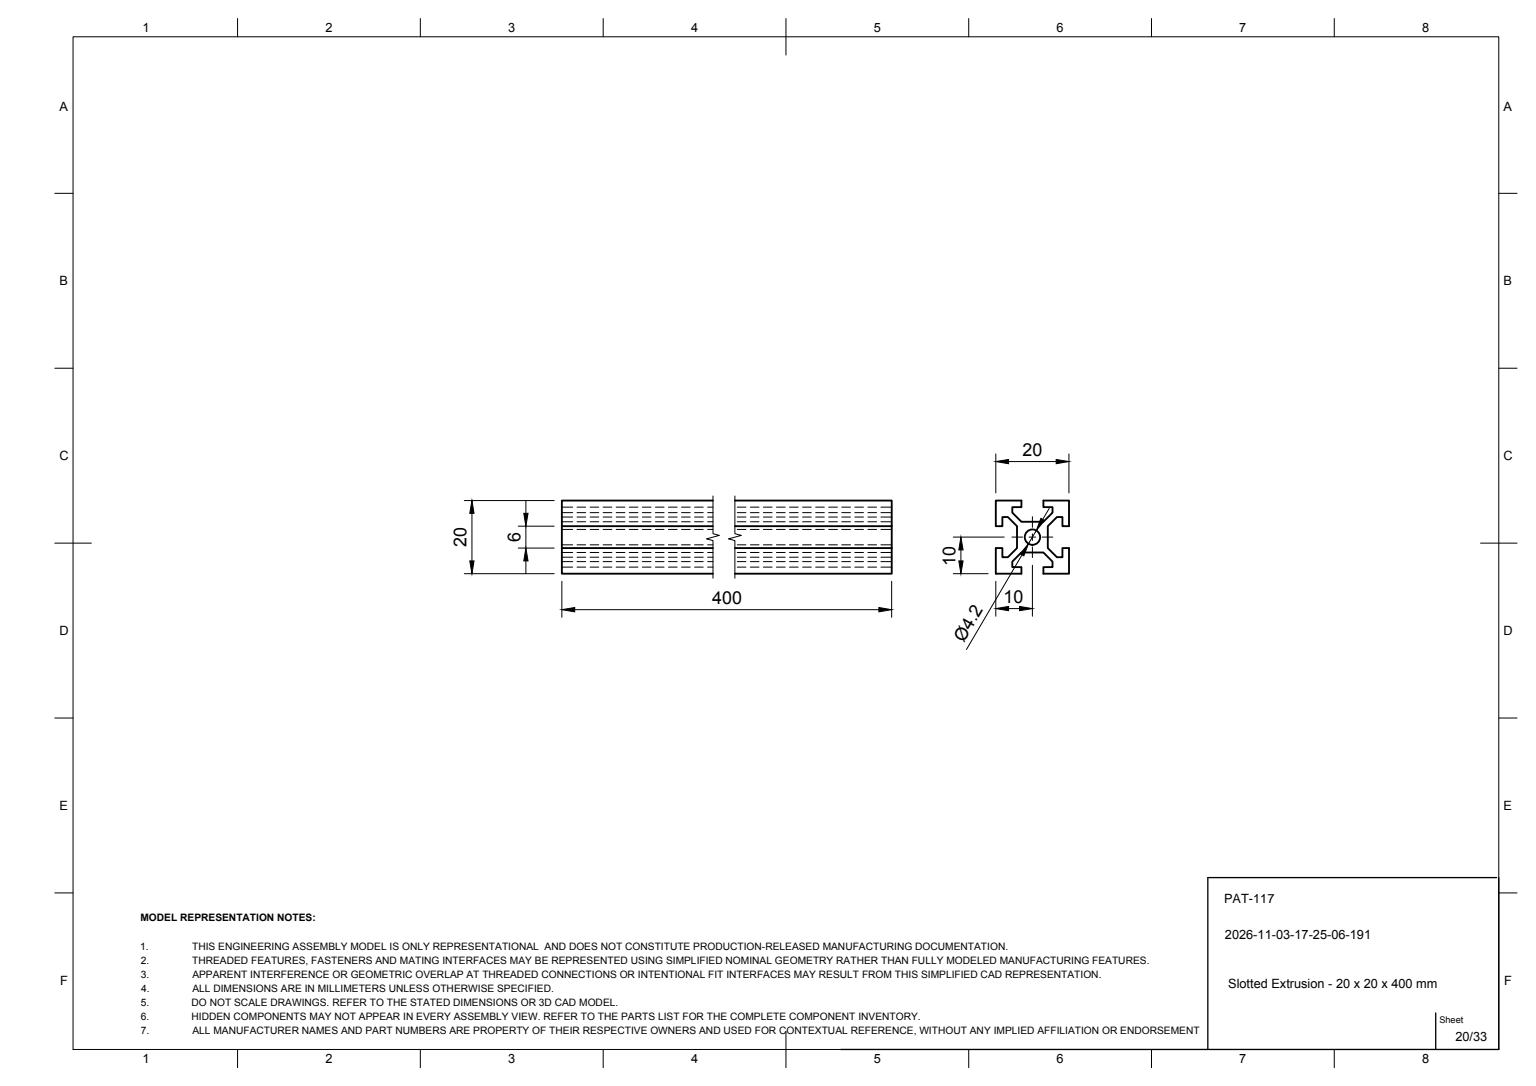
ISO-10303-21;
HEADER;
/* Generated by software containing ST-Developer
 * from STEP Tools, Inc. (www.steptools.com) 
 */

FILE_DESCRIPTION(
/* description */ ('Counterbalanced vertical column'),
/* implementation_level */ '2;1');

FILE_NAME(
/* name */ 'Slotted Extrusion - 20 x 20 x 400 mm.step',
/* time_stamp */ '2026-10-29T16:47:22-07:00',
/* author */ (''),
/* organization */ (''),
/* preprocessor_version */ 'ST-DEVELOPER v20.2',
/* originating_system */ 'Autodesk Translation Framework v15.17.0.0',
/* authorisation */ '');

FILE_SCHEMA (('AUTOMOTIVE_DESIGN { 1 0 10303 214 3 1 1 }'));
ENDSEC;

DATA;
#10=MECHANICAL_DESIGN_GEOMETRIC_PRESENTATION_REPRESENTATION('',(#367),#15040);
#297=SHAPE_REPRESENTATION_RELATIONSHIP('SRR','None',#15201,#332);
#332=ADVANCED_BREP_SHAPE_REPRESENTATION('',(#402),#15020);
#367=STYLED_ITEM('',(#15443),#402);
#402=MANIFOLD_SOLID_BREP('Body1',#7090);
#478=FACE_BOUND('',#1475,.T.);
#479=FACE_BOUND('',#1477,.T.);
#619=PLANE('',#7753);
#620=PLANE('',#7754);
#621=PLANE('',#7755);
#622=PLANE('',#7756);
#623=PLANE('',#7757);
#624=PLANE('',#7758);
#625=PLANE('',#7759);
#626=PLANE('',#7760);
#627=PLANE('',#7761);
#628=PLANE('',#7762);
#629=PLANE('',#7763);
#630=PLANE('',#7764);
#631=PLANE('',#7765);
#632=PLANE('',#7766);
#633=PLANE('',#7767);
#634=PLANE('',#7768);
#635=PLANE('',#7769);
#636=PLANE('',#7770);
#637=PLANE('',#7771);
#638=PLANE('',#7772);
#639=PLANE('',#7773);
#640=PLANE('',#7774);
#641=PLANE('',#7775);
#642=PLANE('',#7776);
#643=PLANE('',#7777);
#644=PLANE('',#7778);
#645=PLANE('',#7779);
#646=PLANE('',#7780);
#647=PLANE('',#7781);
#648=PLANE('',#7782);
#649=PLANE('',#7783);
#650=PLANE('',#7784);
#651=PLANE('',#7785);
#652=PLANE('',#7786);
#653=PLANE('',#7787);
#654=PLANE('',#7788);
#655=PLANE('',#7792);
#656=PLANE('',#7793);
#657=PLANE('',#7794);
#658=PLANE('',#7795);
#659=PLANE('',#7796);
#660=PLANE('',#7797);
#661=PLANE('',#7798);
#662=PLANE('',#7799);
#663=PLANE('',#7800);
#664=PLANE('',#7801);
#962=FACE_OUTER_BOUND('',#1429,.T.);
#963=FACE_OUTER_BOUND('',#1430,.T.);
#964=FACE_OUTER_BOUND('',#1431,.T.);
#965=FACE_OUTER_BOUND('',#1432,.T.);
#966=FACE_OUTER_BOUND('',#1433,.T.);
#967=FACE_OUTER_BOUND('',#1434,.T.);
#968=FACE_OUTER_BOUND('',#1435,.T.);
#969=FACE_OUTER_BOUND('',#1436,.T.);
#970=FACE_OUTER_BOUND('',#1437,.T.);
#971=FACE_OUTER_BOUND('',#1438,.T.);
#972=FACE_OUTER_BOUND('',#1439,.T.);
#973=FACE_OUTER_BOUND('',#1440,.T.);
#974=FACE_OUTER_BOUND('',#1441,.T.);
#975=FACE_OUTER_BOUND('',#1442,.T.);
#976=FACE_OUTER_BOUND('',#1443,.T.);
#977=FACE_OUTER_BOUND('',#1444,.T.);
#978=FACE_OUTER_BOUND('',#1445,.T.);
#979=FACE_OUTER_BOUND('',#1446,.T.);
#980=FACE_OUTER_BOUND('',#1447,.T.);
#981=FACE_OUTER_BOUND('',#1448,.T.);
#982=FACE_OUTER_BOUND('',#1449,.T.);
#983=FACE_OUTER_BOUND('',#1450,.T.);
#984=FACE_OUTER_BOUND('',#1451,.T.);
#985=FACE_OUTER_BOUND('',#1452,.T.);
#986=FACE_OUTER_BOUND('',#1453,.T.);
#987=FACE_OUTER_BOUND('',#1454,.T.);
#988=FACE_OUTER_BOUND('',#1455,.T.);
#989=FACE_OUTER_BOUND('',#1456,.T.);
#990=FACE_OUTER_BOUND('',#1457,.T.);
#991=FACE_OUTER_BOUND('',#1458,.T.);
#992=FACE_OUTER_BOUND('',#1459,.T.);
#993=FACE_OUTER_BOUND('',#1460,.T.);
#994=FACE_OUTER_BOUND('',#1461,.T.);
#995=FACE_OUTER_BOUND('',#1462,.T.);
#996=FACE_OUTER_BOUND('',#1463,.T.);
#997=FACE_OUTER_BOUND('',#1464,.T.);
#998=FACE_OUTER_BOUND('',#1465,.T.);
#999=FACE_OUTER_BOUND('',#1466,.T.);
#1000=FACE_OUTER_BOUND('',#1467,.T.);
#1001=FACE_OUTER_BOUND('',#1468,.T.);
#1002=FACE_OUTER_BOUND('',#1469,.T.);
#1003=FACE_OUTER_BOUND('',#1470,.T.);
#1004=FACE_OUTER_BOUND('',#1471,.T.);
#1005=FACE_OUTER_BOUND('',#1472,.T.);
#1006=FACE_OUTER_BOUND('',#1473,.T.);
#1007=FACE_OUTER_BOUND('',#1474,.T.);
#1008=FACE_OUTER_BOUND('',#1476,.T.);
#1429=EDGE_LOOP('',(#5316,#5317,#5318,#5319));
#1430=EDGE_LOOP('',(#5320,#5321,#5322,#5323));
#1431=EDGE_LOOP('',(#5324,#5325,#5326,#5327));
#1432=EDGE_LOOP('',(#5328,#5329,#5330,#5331));
#1433=EDGE_LOOP('',(#5332,#5333,#5334,#5335));
#1434=EDGE_LOOP('',(#5336,#5337,#5338,#5339));
#1435=EDGE_LOOP('',(#5340,#5341,#5342,#5343));
#1436=EDGE_LOOP('',(#5344,#5345,#5346,#5347));
#1437=EDGE_LOOP('',(#5348,#5349,#5350,#5351));
#1438=EDGE_LOOP('',(#5352,#5353,#5354,#5355));
#1439=EDGE_LOOP('',(#5356,#5357,#5358,#5359));
#1440=EDGE_LOOP('',(#5360,#5361,#5362,#5363));
#1441=EDGE_LOOP('',(#5364,#5365,#5366,#5367));
#1442=EDGE_LOOP('',(#5368,#5369,#5370,#5371));
#1443=EDGE_LOOP('',(#5372,#5373,#5374,#5375));
#1444=EDGE_LOOP('',(#5376,#5377,#5378,#5379));
#1445=EDGE_LOOP('',(#5380,#5381,#5382,#5383));
#1446=EDGE_LOOP('',(#5384,#5385,#5386,#5387));
#1447=EDGE_LOOP('',(#5388,#5389,#5390,#5391));
#1448=EDGE_LOOP('',(#5392,#5393,#5394,#5395));
#1449=EDGE_LOOP('',(#5396,#5397,#5398,#5399));
#1450=EDGE_LOOP('',(#5400,#5401,#5402,#5403));
#1451=EDGE_LOOP('',(#5404,#5405,#5406,#5407));
#1452=EDGE_LOOP('',(#5408,#5409,#5410,#5411));
#1453=EDGE_LOOP('',(#5412,#5413,#5414,#5415));
#1454=EDGE_LOOP('',(#5416,#5417,#5418,#5419));
#1455=EDGE_LOOP('',(#5420,#5421,#5422,#5423));
#1456=EDGE_LOOP('',(#5424,#5425,#5426,#5427));
#1457=EDGE_LOOP('',(#5428,#5429,#5430,#5431));
#1458=EDGE_LOOP('',(#5432,#5433,#5434,#5435));
#1459=EDGE_LOOP('',(#5436,#5437,#5438,#5439));
#1460=EDGE_LOOP('',(#5440,#5441,#5442,#5443));
#1461=EDGE_LOOP('',(#5444,#5445,#5446,#5447));
#1462=EDGE_LOOP('',(#5448,#5449,#5450,#5451));
#1463=EDGE_LOOP('',(#5452,#5453,#5454,#5455));
#1464=EDGE_LOOP('',(#5456,#5457,#5458,#5459));
#1465=EDGE_LOOP('',(#5460,#5461,#5462,#5463));
#1466=EDGE_LOOP('',(#5464,#5465,#5466,#5467));
#1467=EDGE_LOOP('',(#5468,#5469,#5470,#5471));
#1468=EDGE_LOOP('',(#5472,#5473,#5474,#5475));
#1469=EDGE_LOOP('',(#5476,#5477,#5478,#5479));
#1470=EDGE_LOOP('',(#5480,#5481,#5482,#5483));
#1471=EDGE_LOOP('',(#5484,#5485,#5486,#5487));
#1472=EDGE_LOOP('',(#5488,#5489,#5490,#5491));
#1473=EDGE_LOOP('',(#5492,#5493,#5494,#5495));
#1474=EDGE_LOOP('',(#5496,#5497,#5498,#5499,#5500,#5501,#5502,#5503,#5504,
#5505,#5506,#5507,#5508,#5509,#5510,#5511,#5512,#5513,#5514,#5515,#5516,
#5517,#5518,#5519,#5520,#5521,#5522,#5523,#5524,#5525,#5526,#5527,#5528,
#5529,#5530,#5531,#5532,#5533,#5534,#5535,#5536,#5537,#5538,#5539));
#1475=EDGE_LOOP('',(#5540));
#1476=EDGE_LOOP('',(#5541,#5542,#5543,#5544,#5545,#5546,#5547,#5548,#5549,
#5550,#5551,#5552,#5553,#5554,#5555,#5556,#5557,#5558,#5559,#5560,#5561,
#5562,#5563,#5564,#5565,#5566,#5567,#5568,#5569,#5570,#5571,#5572,#5573,
#5574,#5575,#5576,#5577,#5578,#5579,#5580,#5581,#5582,#5583,#5584));
#1477=EDGE_LOOP('',(#5585));
#1914=LINE('',#13575,#2585);
#1915=LINE('',#13577,#2586);
#1916=LINE('',#13579,#2587);
#1917=LINE('',#13580,#2588);
#1918=LINE('',#13583,#2589);
#1919=LINE('',#13585,#2590);
#1920=LINE('',#13586,#2591);
#1921=LINE('',#13589,#2592);
#1922=LINE('',#13591,#2593);
#1923=LINE('',#13592,#2594);
#1924=LINE('',#13595,#2595);
#1925=LINE('',#13597,#2596);
#1926=LINE('',#13598,#2597);
#1927=LINE('',#13601,#2598);
#1928=LINE('',#13603,#2599);
#1929=LINE('',#13604,#2600);
#1930=LINE('',#13607,#2601);
#1931=LINE('',#13609,#2602);
#1932=LINE('',#13610,#2603);
#1933=LINE('',#13613,#2604);
#1934=LINE('',#13615,#2605);
#1935=LINE('',#13616,#2606);
#1936=LINE('',#13619,#2607);
#1937=LINE('',#13621,#2608);
#1938=LINE('',#13622,#2609);
#1939=LINE('',#13625,#2610);
#1940=LINE('',#13627,#2611);
#1941=LINE('',#13628,#2612);
#1942=LINE('',#13632,#2613);
#1943=LINE('',#13634,#2614);
#1944=LINE('',#13636,#2615);
#1945=LINE('',#13637,#2616);
#1946=LINE('',#13640,#2617);
#1947=LINE('',#13642,#2618);
#1948=LINE('',#13643,#2619);
#1949=LINE('',#13646,#2620);
#1950=LINE('',#13648,#2621);
#1951=LINE('',#13649,#2622);
#1952=LINE('',#13652,#2623);
#1953=LINE('',#13654,#2624);
#1954=LINE('',#13655,#2625);
#1955=LINE('',#13658,#2626);
#1956=LINE('',#13660,#2627);
#1957=LINE('',#13661,#2628);
#1958=LINE('',#13664,#2629);
#1959=LINE('',#13666,#2630);
#1960=LINE('',#13667,#2631);
#1961=LINE('',#13670,#2632);
#1962=LINE('',#13672,#2633);
#1963=LINE('',#13673,#2634);
#1964=LINE('',#13676,#2635);
#1965=LINE('',#13678,#2636);
#1966=LINE('',#13679,#2637);
#1967=LINE('',#13682,#2638);
#1968=LINE('',#13684,#2639);
#1969=LINE('',#13685,#2640);
#1970=LINE('',#13689,#2641);
#1971=LINE('',#13691,#2642);
#1972=LINE('',#13693,#2643);
#1973=LINE('',#13694,#2644);
#1974=LINE('',#13697,#2645);
#1975=LINE('',#13699,#2646);
#1976=LINE('',#13700,#2647);
#1977=LINE('',#13703,#2648);
#1978=LINE('',#13705,#2649);
#1979=LINE('',#13706,#2650);
#1980=LINE('',#13709,#2651);
#1981=LINE('',#13711,#2652);
#1982=LINE('',#13712,#2653);
#1983=LINE('',#13715,#2654);
#1984=LINE('',#13717,#2655);
#1985=LINE('',#13718,#2656);
#1986=LINE('',#13721,#2657);
#1987=LINE('',#13723,#2658);
#1988=LINE('',#13724,#2659);
#1989=LINE('',#13727,#2660);
#1990=LINE('',#13729,#2661);
#1991=LINE('',#13730,#2662);
#1992=LINE('',#13733,#2663);
#1993=LINE('',#13735,#2664);
#1994=LINE('',#13736,#2665);
#1995=LINE('',#13739,#2666);
#1996=LINE('',#13741,#2667);
#1997=LINE('',#13742,#2668);
#1998=LINE('',#13746,#2669);
#1999=LINE('',#13748,#2670);
#2000=LINE('',#13750,#2671);
#2001=LINE('',#13751,#2672);
#2002=LINE('',#13754,#2673);
#2003=LINE('',#13756,#2674);
#2004=LINE('',#13757,#2675);
#2005=LINE('',#13760,#2676);
#2006=LINE('',#13762,#2677);
#2007=LINE('',#13763,#2678);
#2008=LINE('',#13766,#2679);
#2009=LINE('',#13768,#2680);
#2010=LINE('',#13769,#2681);
#2011=LINE('',#13772,#2682);
#2012=LINE('',#13774,#2683);
#2013=LINE('',#13775,#2684);
#2014=LINE('',#13778,#2685);
#2015=LINE('',#13780,#2686);
#2016=LINE('',#13781,#2687);
#2017=LINE('',#13784,#2688);
#2018=LINE('',#13786,#2689);
#2019=LINE('',#13787,#2690);
#2020=LINE('',#13790,#2691);
#2021=LINE('',#13792,#2692);
#2022=LINE('',#13793,#2693);
#2023=LINE('',#13796,#2694);
#2024=LINE('',#13798,#2695);
#2025=LINE('',#13799,#2696);
#2026=LINE('',#13804,#2697);
#2027=LINE('',#13808,#2698);
#2028=LINE('',#13810,#2699);
#2029=LINE('',#13811,#2700);
#2030=LINE('',#13814,#2701);
#2031=LINE('',#13816,#2702);
#2032=LINE('',#13817,#2703);
#2033=LINE('',#13819,#2704);
#2034=LINE('',#13820,#2705);
#2035=LINE('',#13823,#2706);
#2036=LINE('',#13825,#2707);
#2037=LINE('',#13826,#2708);
#2038=LINE('',#13828,#2709);
#2039=LINE('',#13829,#2710);
#2040=LINE('',#13832,#2711);
#2041=LINE('',#13834,#2712);
#2042=LINE('',#13835,#2713);
#2043=LINE('',#13837,#2714);
#2044=LINE('',#13838,#2715);
#2045=LINE('',#13840,#2716);
#2046=LINE('',#13841,#2717);
#2585=VECTOR('',#8896,1.);
#2586=VECTOR('',#8897,1.);
#2587=VECTOR('',#8898,1.);
#2588=VECTOR('',#8899,1.);
#2589=VECTOR('',#8902,1.);
#2590=VECTOR('',#8903,1.);
#2591=VECTOR('',#8904,1.);
#2592=VECTOR('',#8907,1.);
#2593=VECTOR('',#8908,1.);
#2594=VECTOR('',#8909,1.);
#2595=VECTOR('',#8912,1.);
#2596=VECTOR('',#8913,1.);
#2597=VECTOR('',#8914,1.);
#2598=VECTOR('',#8917,1.);
#2599=VECTOR('',#8918,1.);
#2600=VECTOR('',#8919,1.);
#2601=VECTOR('',#8922,1.);
#2602=VECTOR('',#8923,1.);
#2603=VECTOR('',#8924,1.);
#2604=VECTOR('',#8927,1.);
#2605=VECTOR('',#8928,1.);
#2606=VECTOR('',#8929,1.);
#2607=VECTOR('',#8932,1.);
#2608=VECTOR('',#8933,1.);
#2609=VECTOR('',#8934,1.);
#2610=VECTOR('',#8937,1.);
#2611=VECTOR('',#8938,1.);
#2612=VECTOR('',#8939,1.);
#2613=VECTOR('',#8942,1.);
#2614=VECTOR('',#8943,1.);
#2615=VECTOR('',#8944,1.);
#2616=VECTOR('',#8945,1.);
#2617=VECTOR('',#8948,1.);
#2618=VECTOR('',#8949,1.);
#2619=VECTOR('',#8950,1.);
#2620=VECTOR('',#8953,1.);
#2621=VECTOR('',#8954,1.);
#2622=VECTOR('',#8955,1.);
#2623=VECTOR('',#8958,1.);
#2624=VECTOR('',#8959,1.);
#2625=VECTOR('',#8960,1.);
#2626=VECTOR('',#8963,1.);
#2627=VECTOR('',#8964,1.);
#2628=VECTOR('',#8965,1.);
#2629=VECTOR('',#8968,1.);
#2630=VECTOR('',#8969,1.);
#2631=VECTOR('',#8970,1.);
#2632=VECTOR('',#8973,1.);
#2633=VECTOR('',#8974,1.);
#2634=VECTOR('',#8975,1.);
#2635=VECTOR('',#8978,1.);
#2636=VECTOR('',#8979,1.);
#2637=VECTOR('',#8980,1.);
#2638=VECTOR('',#8983,1.);
#2639=VECTOR('',#8984,1.);
#2640=VECTOR('',#8985,1.);
#2641=VECTOR('',#8988,1.);
#2642=VECTOR('',#8989,1.);
#2643=VECTOR('',#8990,1.);
#2644=VECTOR('',#8991,1.);
#2645=VECTOR('',#8994,1.);
#2646=VECTOR('',#8995,1.);
#2647=VECTOR('',#8996,1.);
#2648=VECTOR('',#8999,1.);
#2649=VECTOR('',#9000,1.);
#2650=VECTOR('',#9001,1.);
#2651=VECTOR('',#9004,1.);
#2652=VECTOR('',#9005,1.);
#2653=VECTOR('',#9006,1.);
#2654=VECTOR('',#9009,1.);
#2655=VECTOR('',#9010,1.);
#2656=VECTOR('',#9011,1.);
#2657=VECTOR('',#9014,1.);
#2658=VECTOR('',#9015,1.);
#2659=VECTOR('',#9016,1.);
#2660=VECTOR('',#9019,1.);
#2661=VECTOR('',#9020,1.);
#2662=VECTOR('',#9021,1.);
#2663=VECTOR('',#9024,1.);
#2664=VECTOR('',#9025,1.);
#2665=VECTOR('',#9026,1.);
#2666=VECTOR('',#9029,1.);
#2667=VECTOR('',#9030,1.);
#2668=VECTOR('',#9031,1.);
#2669=VECTOR('',#9034,1.);
#2670=VECTOR('',#9035,1.);
#2671=VECTOR('',#9036,1.);
#2672=VECTOR('',#9037,1.);
#2673=VECTOR('',#9040,1.);
#2674=VECTOR('',#9041,1.);
#2675=VECTOR('',#9042,1.);
#2676=VECTOR('',#9045,1.);
#2677=VECTOR('',#9046,1.);
#2678=VECTOR('',#9047,1.);
#2679=VECTOR('',#9050,1.);
#2680=VECTOR('',#9051,1.);
#2681=VECTOR('',#9052,1.);
#2682=VECTOR('',#9055,1.);
#2683=VECTOR('',#9056,1.);
#2684=VECTOR('',#9057,1.);
#2685=VECTOR('',#9060,1.);
#2686=VECTOR('',#9061,1.);
#2687=VECTOR('',#9062,1.);
#2688=VECTOR('',#9065,1.);
#2689=VECTOR('',#9066,1.);
#2690=VECTOR('',#9067,1.);
#2691=VECTOR('',#9070,1.);
#2692=VECTOR('',#9071,1.);
#2693=VECTOR('',#9072,1.);
#2694=VECTOR('',#9075,1.);
#2695=VECTOR('',#9076,1.);
#2696=VECTOR('',#9077,1.);
#2697=VECTOR('',#9082,0.21);
#2698=VECTOR('',#9087,1.);
#2699=VECTOR('',#9088,1.);
#2700=VECTOR('',#9089,1.);
#2701=VECTOR('',#9092,1.);
#2702=VECTOR('',#9093,1.);
#2703=VECTOR('',#9094,1.);
#2704=VECTOR('',#9097,1.);
#2705=VECTOR('',#9098,1.);
#2706=VECTOR('',#9101,1.);
#2707=VECTOR('',#9102,1.);
#2708=VECTOR('',#9103,1.);
#2709=VECTOR('',#9106,1.);
#2710=VECTOR('',#9107,1.);
#2711=VECTOR('',#9110,1.);
#2712=VECTOR('',#9111,1.);
#2713=VECTOR('',#9112,1.);
#2714=VECTOR('',#9115,1.);
#2715=VECTOR('',#9116,1.);
#2716=VECTOR('',#9119,1.);
#2717=VECTOR('',#9120,1.);
#3187=CIRCLE('',#7790,0.21);
#3188=CIRCLE('',#7791,0.21);
#3482=VERTEX_POINT('',#13573);
#3483=VERTEX_POINT('',#13574);
#3484=VERTEX_POINT('',#13576);
#3485=VERTEX_POINT('',#13578);
#3486=VERTEX_POINT('',#13582);
#3487=VERTEX_POINT('',#13584);
#3488=VERTEX_POINT('',#13588);
#3489=VERTEX_POINT('',#13590);
#3490=VERTEX_POINT('',#13594);
#3491=VERTEX_POINT('',#13596);
#3492=VERTEX_POINT('',#13600);
#3493=VERTEX_POINT('',#13602);
#3494=VERTEX_POINT('',#13606);
#3495=VERTEX_POINT('',#13608);
#3496=VERTEX_POINT('',#13612);
#3497=VERTEX_POINT('',#13614);
#3498=VERTEX_POINT('',#13618);
#3499=VERTEX_POINT('',#13620);
#3500=VERTEX_POINT('',#13624);
#3501=VERTEX_POINT('',#13626);
#3502=VERTEX_POINT('',#13630);
#3503=VERTEX_POINT('',#13631);
#3504=VERTEX_POINT('',#13633);
#3505=VERTEX_POINT('',#13635);
#3506=VERTEX_POINT('',#13639);
#3507=VERTEX_POINT('',#13641);
#3508=VERTEX_POINT('',#13645);
#3509=VERTEX_POINT('',#13647);
#3510=VERTEX_POINT('',#13651);
#3511=VERTEX_POINT('',#13653);
#3512=VERTEX_POINT('',#13657);
#3513=VERTEX_POINT('',#13659);
#3514=VERTEX_POINT('',#13663);
#3515=VERTEX_POINT('',#13665);
#3516=VERTEX_POINT('',#13669);
#3517=VERTEX_POINT('',#13671);
#3518=VERTEX_POINT('',#13675);
#3519=VERTEX_POINT('',#13677);
#3520=VERTEX_POINT('',#13681);
#3521=VERTEX_POINT('',#13683);
#3522=VERTEX_POINT('',#13687);
#3523=VERTEX_POINT('',#13688);
#3524=VERTEX_POINT('',#13690);
#3525=VERTEX_POINT('',#13692);
#3526=VERTEX_POINT('',#13696);
#3527=VERTEX_POINT('',#13698);
#3528=VERTEX_POINT('',#13702);
#3529=VERTEX_POINT('',#13704);
#3530=VERTEX_POINT('',#13708);
#3531=VERTEX_POINT('',#13710);
#3532=VERTEX_POINT('',#13714);
#3533=VERTEX_POINT('',#13716);
#3534=VERTEX_POINT('',#13720);
#3535=VERTEX_POINT('',#13722);
#3536=VERTEX_POINT('',#13726);
#3537=VERTEX_POINT('',#13728);
#3538=VERTEX_POINT('',#13732);
#3539=VERTEX_POINT('',#13734);
#3540=VERTEX_POINT('',#13738);
#3541=VERTEX_POINT('',#13740);
#3542=VERTEX_POINT('',#13744);
#3543=VERTEX_POINT('',#13745);
#3544=VERTEX_POINT('',#13747);
#3545=VERTEX_POINT('',#13749);
#3546=VERTEX_POINT('',#13753);
#3547=VERTEX_POINT('',#13755);
#3548=VERTEX_POINT('',#13759);
#3549=VERTEX_POINT('',#13761);
#3550=VERTEX_POINT('',#13765);
#3551=VERTEX_POINT('',#13767);
#3552=VERTEX_POINT('',#13771);
#3553=VERTEX_POINT('',#13773);
#3554=VERTEX_POINT('',#13777);
#3555=VERTEX_POINT('',#13779);
#3556=VERTEX_POINT('',#13783);
#3557=VERTEX_POINT('',#13785);
#3558=VERTEX_POINT('',#13789);
#3559=VERTEX_POINT('',#13791);
#3560=VERTEX_POINT('',#13795);
#3561=VERTEX_POINT('',#13797);
#3562=VERTEX_POINT('',#13801);
#3563=VERTEX_POINT('',#13803);
#3564=VERTEX_POINT('',#13807);
#3565=VERTEX_POINT('',#13809);
#3566=VERTEX_POINT('',#13813);
#3567=VERTEX_POINT('',#13815);
#3568=VERTEX_POINT('',#13822);
#3569=VERTEX_POINT('',#13824);
#3570=VERTEX_POINT('',#13831);
#3571=VERTEX_POINT('',#13833);
#4159=EDGE_CURVE('',#3482,#3483,#1914,.T.);
#4160=EDGE_CURVE('',#3482,#3484,#1915,.T.);
#4161=EDGE_CURVE('',#3485,#3484,#1916,.T.);
#4162=EDGE_CURVE('',#3483,#3485,#1917,.T.);
#4163=EDGE_CURVE('',#3486,#3482,#1918,.T.);
#4164=EDGE_CURVE('',#3486,#3487,#1919,.T.);
#4165=EDGE_CURVE('',#3484,#3487,#1920,.T.);
#4166=EDGE_CURVE('',#3488,#3486,#1921,.T.);
#4167=EDGE_CURVE('',#3488,#3489,#1922,.T.);
#4168=EDGE_CURVE('',#3487,#3489,#1923,.T.);
#4169=EDGE_CURVE('',#3490,#3488,#1924,.T.);
#4170=EDGE_CURVE('',#3490,#3491,#1925,.T.);
#4171=EDGE_CURVE('',#3489,#3491,#1926,.T.);
#4172=EDGE_CURVE('',#3492,#3490,#1927,.T.);
#4173=EDGE_CURVE('',#3492,#3493,#1928,.T.);
#4174=EDGE_CURVE('',#3491,#3493,#1929,.T.);
#4175=EDGE_CURVE('',#3494,#3492,#1930,.T.);
#4176=EDGE_CURVE('',#3494,#3495,#1931,.T.);
#4177=EDGE_CURVE('',#3493,#3495,#1932,.T.);
#4178=EDGE_CURVE('',#3496,#3494,#1933,.T.);
#4179=EDGE_CURVE('',#3496,#3497,#1934,.T.);
#4180=EDGE_CURVE('',#3495,#3497,#1935,.T.);
#4181=EDGE_CURVE('',#3498,#3496,#1936,.T.);
#4182=EDGE_CURVE('',#3498,#3499,#1937,.T.);
#4183=EDGE_CURVE('',#3497,#3499,#1938,.T.);
#4184=EDGE_CURVE('',#3500,#3498,#1939,.T.);
#4185=EDGE_CURVE('',#3501,#3500,#1940,.T.);
#4186=EDGE_CURVE('',#3499,#3501,#1941,.T.);
#4187=EDGE_CURVE('',#3502,#3503,#1942,.T.);
#4188=EDGE_CURVE('',#3502,#3504,#1943,.T.);
#4189=EDGE_CURVE('',#3505,#3504,#1944,.T.);
#4190=EDGE_CURVE('',#3503,#3505,#1945,.T.);
#4191=EDGE_CURVE('',#3506,#3502,#1946,.T.);
#4192=EDGE_CURVE('',#3506,#3507,#1947,.T.);
#4193=EDGE_CURVE('',#3504,#3507,#1948,.T.);
#4194=EDGE_CURVE('',#3508,#3506,#1949,.T.);
#4195=EDGE_CURVE('',#3508,#3509,#1950,.T.);
#4196=EDGE_CURVE('',#3507,#3509,#1951,.T.);
#4197=EDGE_CURVE('',#3510,#3508,#1952,.T.);
#4198=EDGE_CURVE('',#3510,#3511,#1953,.T.);
#4199=EDGE_CURVE('',#3509,#3511,#1954,.T.);
#4200=EDGE_CURVE('',#3512,#3510,#1955,.T.);
#4201=EDGE_CURVE('',#3512,#3513,#1956,.T.);
#4202=EDGE_CURVE('',#3511,#3513,#1957,.T.);
#4203=EDGE_CURVE('',#3514,#3512,#1958,.T.);
#4204=EDGE_CURVE('',#3514,#3515,#1959,.T.);
#4205=EDGE_CURVE('',#3513,#3515,#1960,.T.);
#4206=EDGE_CURVE('',#3516,#3514,#1961,.T.);
#4207=EDGE_CURVE('',#3516,#3517,#1962,.T.);
#4208=EDGE_CURVE('',#3515,#3517,#1963,.T.);
#4209=EDGE_CURVE('',#3518,#3516,#1964,.T.);
#4210=EDGE_CURVE('',#3518,#3519,#1965,.T.);
#4211=EDGE_CURVE('',#3517,#3519,#1966,.T.);
#4212=EDGE_CURVE('',#3520,#3518,#1967,.T.);
#4213=EDGE_CURVE('',#3521,#3520,#1968,.T.);
#4214=EDGE_CURVE('',#3519,#3521,#1969,.T.);
#4215=EDGE_CURVE('',#3522,#3523,#1970,.T.);
#4216=EDGE_CURVE('',#3522,#3524,#1971,.T.);
#4217=EDGE_CURVE('',#3525,#3524,#1972,.T.);
#4218=EDGE_CURVE('',#3523,#3525,#1973,.T.);
#4219=EDGE_CURVE('',#3526,#3522,#1974,.T.);
#4220=EDGE_CURVE('',#3526,#3527,#1975,.T.);
#4221=EDGE_CURVE('',#3524,#3527,#1976,.T.);
#4222=EDGE_CURVE('',#3528,#3526,#1977,.T.);
#4223=EDGE_CURVE('',#3528,#3529,#1978,.T.);
#4224=EDGE_CURVE('',#3527,#3529,#1979,.T.);
#4225=EDGE_CURVE('',#3530,#3528,#1980,.T.);
#4226=EDGE_CURVE('',#3530,#3531,#1981,.T.);
#4227=EDGE_CURVE('',#3529,#3531,#1982,.T.);
#4228=EDGE_CURVE('',#3532,#3530,#1983,.T.);
#4229=EDGE_CURVE('',#3532,#3533,#1984,.T.);
#4230=EDGE_CURVE('',#3531,#3533,#1985,.T.);
#4231=EDGE_CURVE('',#3534,#3532,#1986,.T.);
#4232=EDGE_CURVE('',#3534,#3535,#1987,.T.);
#4233=EDGE_CURVE('',#3533,#3535,#1988,.T.);
#4234=EDGE_CURVE('',#3536,#3534,#1989,.T.);
#4235=EDGE_CURVE('',#3536,#3537,#1990,.T.);
#4236=EDGE_CURVE('',#3535,#3537,#1991,.T.);
#4237=EDGE_CURVE('',#3538,#3536,#1992,.T.);
#4238=EDGE_CURVE('',#3538,#3539,#1993,.T.);
#4239=EDGE_CURVE('',#3537,#3539,#1994,.T.);
#4240=EDGE_CURVE('',#3540,#3538,#1995,.T.);
#4241=EDGE_CURVE('',#3541,#3540,#1996,.T.);
#4242=EDGE_CURVE('',#3539,#3541,#1997,.T.);
#4243=EDGE_CURVE('',#3542,#3543,#1998,.T.);
#4244=EDGE_CURVE('',#3542,#3544,#1999,.T.);
#4245=EDGE_CURVE('',#3545,#3544,#2000,.T.);
#4246=EDGE_CURVE('',#3543,#3545,#2001,.T.);
#4247=EDGE_CURVE('',#3546,#3542,#2002,.T.);
#4248=EDGE_CURVE('',#3546,#3547,#2003,.T.);
#4249=EDGE_CURVE('',#3544,#3547,#2004,.T.);
#4250=EDGE_CURVE('',#3548,#3546,#2005,.T.);
#4251=EDGE_CURVE('',#3548,#3549,#2006,.T.);
#4252=EDGE_CURVE('',#3547,#3549,#2007,.T.);
#4253=EDGE_CURVE('',#3550,#3548,#2008,.T.);
#4254=EDGE_CURVE('',#3550,#3551,#2009,.T.);
#4255=EDGE_CURVE('',#3549,#3551,#2010,.T.);
#4256=EDGE_CURVE('',#3552,#3550,#2011,.T.);
#4257=EDGE_CURVE('',#3552,#3553,#2012,.T.);
#4258=EDGE_CURVE('',#3551,#3553,#2013,.T.);
#4259=EDGE_CURVE('',#3554,#3552,#2014,.T.);
#4260=EDGE_CURVE('',#3554,#3555,#2015,.T.);
#4261=EDGE_CURVE('',#3553,#3555,#2016,.T.);
#4262=EDGE_CURVE('',#3556,#3554,#2017,.T.);
#4263=EDGE_CURVE('',#3556,#3557,#2018,.T.);
#4264=EDGE_CURVE('',#3555,#3557,#2019,.T.);
#4265=EDGE_CURVE('',#3558,#3556,#2020,.T.);
#4266=EDGE_CURVE('',#3558,#3559,#2021,.T.);
#4267=EDGE_CURVE('',#3557,#3559,#2022,.T.);
#4268=EDGE_CURVE('',#3560,#3558,#2023,.T.);
#4269=EDGE_CURVE('',#3561,#3560,#2024,.T.);
#4270=EDGE_CURVE('',#3559,#3561,#2025,.T.);
#4271=EDGE_CURVE('',#3562,#3562,#3187,.T.);
#4272=EDGE_CURVE('',#3562,#3563,#2026,.T.);
#4273=EDGE_CURVE('',#3563,#3563,#3188,.T.);
#4274=EDGE_CURVE('',#3500,#3564,#2027,.T.);
#4275=EDGE_CURVE('',#3564,#3565,#2028,.T.);
#4276=EDGE_CURVE('',#3501,#3565,#2029,.T.);
#4277=EDGE_CURVE('',#3566,#3485,#2030,.T.);
#4278=EDGE_CURVE('',#3567,#3566,#2031,.T.);
#4279=EDGE_CURVE('',#3567,#3483,#2032,.T.);
#4280=EDGE_CURVE('',#3520,#3567,#2033,.T.);
#4281=EDGE_CURVE('',#3521,#3566,#2034,.T.);
#4282=EDGE_CURVE('',#3568,#3505,#2035,.T.);
#4283=EDGE_CURVE('',#3569,#3568,#2036,.T.);
#4284=EDGE_CURVE('',#3569,#3503,#2037,.T.);
#4285=EDGE_CURVE('',#3540,#3569,#2038,.T.);
#4286=EDGE_CURVE('',#3541,#3568,#2039,.T.);
#4287=EDGE_CURVE('',#3570,#3525,#2040,.T.);
#4288=EDGE_CURVE('',#3571,#3570,#2041,.T.);
#4289=EDGE_CURVE('',#3571,#3523,#2042,.T.);
#4290=EDGE_CURVE('',#3560,#3571,#2043,.T.);
#4291=EDGE_CURVE('',#3561,#3570,#2044,.T.);
#4292=EDGE_CURVE('',#3565,#3545,#2045,.T.);
#4293=EDGE_CURVE('',#3564,#3543,#2046,.T.);
#5316=ORIENTED_EDGE('',*,*,#4159,.F.);
#5317=ORIENTED_EDGE('',*,*,#4160,.T.);
#5318=ORIENTED_EDGE('',*,*,#4161,.F.);
#5319=ORIENTED_EDGE('',*,*,#4162,.F.);
#5320=ORIENTED_EDGE('',*,*,#4163,.F.);
#5321=ORIENTED_EDGE('',*,*,#4164,.T.);
#5322=ORIENTED_EDGE('',*,*,#4165,.F.);
#5323=ORIENTED_EDGE('',*,*,#4160,.F.);
#5324=ORIENTED_EDGE('',*,*,#4166,.F.);
#5325=ORIENTED_EDGE('',*,*,#4167,.T.);
#5326=ORIENTED_EDGE('',*,*,#4168,.F.);
#5327=ORIENTED_EDGE('',*,*,#4164,.F.);
#5328=ORIENTED_EDGE('',*,*,#4169,.F.);
#5329=ORIENTED_EDGE('',*,*,#4170,.T.);
#5330=ORIENTED_EDGE('',*,*,#4171,.F.);
#5331=ORIENTED_EDGE('',*,*,#4167,.F.);
#5332=ORIENTED_EDGE('',*,*,#4172,.F.);
#5333=ORIENTED_EDGE('',*,*,#4173,.T.);
#5334=ORIENTED_EDGE('',*,*,#4174,.F.);
#5335=ORIENTED_EDGE('',*,*,#4170,.F.);
#5336=ORIENTED_EDGE('',*,*,#4175,.F.);
#5337=ORIENTED_EDGE('',*,*,#4176,.T.);
#5338=ORIENTED_EDGE('',*,*,#4177,.F.);
#5339=ORIENTED_EDGE('',*,*,#4173,.F.);
#5340=ORIENTED_EDGE('',*,*,#4178,.F.);
#5341=ORIENTED_EDGE('',*,*,#4179,.T.);
#5342=ORIENTED_EDGE('',*,*,#4180,.F.);
#5343=ORIENTED_EDGE('',*,*,#4176,.F.);
#5344=ORIENTED_EDGE('',*,*,#4181,.F.);
#5345=ORIENTED_EDGE('',*,*,#4182,.T.);
#5346=ORIENTED_EDGE('',*,*,#4183,.F.);
#5347=ORIENTED_EDGE('',*,*,#4179,.F.);
#5348=ORIENTED_EDGE('',*,*,#4184,.F.);
#5349=ORIENTED_EDGE('',*,*,#4185,.F.);
#5350=ORIENTED_EDGE('',*,*,#4186,.F.);
#5351=ORIENTED_EDGE('',*,*,#4182,.F.);
#5352=ORIENTED_EDGE('',*,*,#4187,.F.);
#5353=ORIENTED_EDGE('',*,*,#4188,.T.);
#5354=ORIENTED_EDGE('',*,*,#4189,.F.);
#5355=ORIENTED_EDGE('',*,*,#4190,.F.);
#5356=ORIENTED_EDGE('',*,*,#4191,.F.);
#5357=ORIENTED_EDGE('',*,*,#4192,.T.);
#5358=ORIENTED_EDGE('',*,*,#4193,.F.);
#5359=ORIENTED_EDGE('',*,*,#4188,.F.);
#5360=ORIENTED_EDGE('',*,*,#4194,.F.);
#5361=ORIENTED_EDGE('',*,*,#4195,.T.);
#5362=ORIENTED_EDGE('',*,*,#4196,.F.);
#5363=ORIENTED_EDGE('',*,*,#4192,.F.);
#5364=ORIENTED_EDGE('',*,*,#4197,.F.);
#5365=ORIENTED_EDGE('',*,*,#4198,.T.);
#5366=ORIENTED_EDGE('',*,*,#4199,.F.);
#5367=ORIENTED_EDGE('',*,*,#4195,.F.);
#5368=ORIENTED_EDGE('',*,*,#4200,.F.);
#5369=ORIENTED_EDGE('',*,*,#4201,.T.);
#5370=ORIENTED_EDGE('',*,*,#4202,.F.);
#5371=ORIENTED_EDGE('',*,*,#4198,.F.);
#5372=ORIENTED_EDGE('',*,*,#4203,.F.);
#5373=ORIENTED_EDGE('',*,*,#4204,.T.);
#5374=ORIENTED_EDGE('',*,*,#4205,.F.);
#5375=ORIENTED_EDGE('',*,*,#4201,.F.);
#5376=ORIENTED_EDGE('',*,*,#4206,.F.);
#5377=ORIENTED_EDGE('',*,*,#4207,.T.);
#5378=ORIENTED_EDGE('',*,*,#4208,.F.);
#5379=ORIENTED_EDGE('',*,*,#4204,.F.);
#5380=ORIENTED_EDGE('',*,*,#4209,.F.);
#5381=ORIENTED_EDGE('',*,*,#4210,.T.);
#5382=ORIENTED_EDGE('',*,*,#4211,.F.);
#5383=ORIENTED_EDGE('',*,*,#4207,.F.);
#5384=ORIENTED_EDGE('',*,*,#4212,.F.);
#5385=ORIENTED_EDGE('',*,*,#4213,.F.);
#5386=ORIENTED_EDGE('',*,*,#4214,.F.);
#5387=ORIENTED_EDGE('',*,*,#4210,.F.);
#5388=ORIENTED_EDGE('',*,*,#4215,.F.);
#5389=ORIENTED_EDGE('',*,*,#4216,.T.);
#5390=ORIENTED_EDGE('',*,*,#4217,.F.);
#5391=ORIENTED_EDGE('',*,*,#4218,.F.);
#5392=ORIENTED_EDGE('',*,*,#4219,.F.);
#5393=ORIENTED_EDGE('',*,*,#4220,.T.);
#5394=ORIENTED_EDGE('',*,*,#4221,.F.);
#5395=ORIENTED_EDGE('',*,*,#4216,.F.);
#5396=ORIENTED_EDGE('',*,*,#4222,.F.);
#5397=ORIENTED_EDGE('',*,*,#4223,.T.);
#5398=ORIENTED_EDGE('',*,*,#4224,.F.);
#5399=ORIENTED_EDGE('',*,*,#4220,.F.);
#5400=ORIENTED_EDGE('',*,*,#4225,.F.);
#5401=ORIENTED_EDGE('',*,*,#4226,.T.);
#5402=ORIENTED_EDGE('',*,*,#4227,.F.);
#5403=ORIENTED_EDGE('',*,*,#4223,.F.);
#5404=ORIENTED_EDGE('',*,*,#4228,.F.);
#5405=ORIENTED_EDGE('',*,*,#4229,.T.);
#5406=ORIENTED_EDGE('',*,*,#4230,.F.);
#5407=ORIENTED_EDGE('',*,*,#4226,.F.);
#5408=ORIENTED_EDGE('',*,*,#4231,.F.);
#5409=ORIENTED_EDGE('',*,*,#4232,.T.);
#5410=ORIENTED_EDGE('',*,*,#4233,.F.);
#5411=ORIENTED_EDGE('',*,*,#4229,.F.);
#5412=ORIENTED_EDGE('',*,*,#4234,.F.);
#5413=ORIENTED_EDGE('',*,*,#4235,.T.);
#5414=ORIENTED_EDGE('',*,*,#4236,.F.);
#5415=ORIENTED_EDGE('',*,*,#4232,.F.);
#5416=ORIENTED_EDGE('',*,*,#4237,.F.);
#5417=ORIENTED_EDGE('',*,*,#4238,.T.);
#5418=ORIENTED_EDGE('',*,*,#4239,.F.);
#5419=ORIENTED_EDGE('',*,*,#4235,.F.);
#5420=ORIENTED_EDGE('',*,*,#4240,.F.);
#5421=ORIENTED_EDGE('',*,*,#4241,.F.);
#5422=ORIENTED_EDGE('',*,*,#4242,.F.);
#5423=ORIENTED_EDGE('',*,*,#4238,.F.);
#5424=ORIENTED_EDGE('',*,*,#4243,.F.);
#5425=ORIENTED_EDGE('',*,*,#4244,.T.);
#5426=ORIENTED_EDGE('',*,*,#4245,.F.);
#5427=ORIENTED_EDGE('',*,*,#4246,.F.);
#5428=ORIENTED_EDGE('',*,*,#4247,.F.);
#5429=ORIENTED_EDGE('',*,*,#4248,.T.);
#5430=ORIENTED_EDGE('',*,*,#4249,.F.);
#5431=ORIENTED_EDGE('',*,*,#4244,.F.);
#5432=ORIENTED_EDGE('',*,*,#4250,.F.);
#5433=ORIENTED_EDGE('',*,*,#4251,.T.);
#5434=ORIENTED_EDGE('',*,*,#4252,.F.);
#5435=ORIENTED_EDGE('',*,*,#4248,.F.);
#5436=ORIENTED_EDGE('',*,*,#4253,.F.);
#5437=ORIENTED_EDGE('',*,*,#4254,.T.);
#5438=ORIENTED_EDGE('',*,*,#4255,.F.);
#5439=ORIENTED_EDGE('',*,*,#4251,.F.);
#5440=ORIENTED_EDGE('',*,*,#4256,.F.);
#5441=ORIENTED_EDGE('',*,*,#4257,.T.);
#5442=ORIENTED_EDGE('',*,*,#4258,.F.);
#5443=ORIENTED_EDGE('',*,*,#4254,.F.);
#5444=ORIENTED_EDGE('',*,*,#4259,.F.);
#5445=ORIENTED_EDGE('',*,*,#4260,.T.);
#5446=ORIENTED_EDGE('',*,*,#4261,.F.);
#5447=ORIENTED_EDGE('',*,*,#4257,.F.);
#5448=ORIENTED_EDGE('',*,*,#4262,.F.);
#5449=ORIENTED_EDGE('',*,*,#4263,.T.);
#5450=ORIENTED_EDGE('',*,*,#4264,.F.);
#5451=ORIENTED_EDGE('',*,*,#4260,.F.);
#5452=ORIENTED_EDGE('',*,*,#4265,.F.);
#5453=ORIENTED_EDGE('',*,*,#4266,.T.);
#5454=ORIENTED_EDGE('',*,*,#4267,.F.);
#5455=ORIENTED_EDGE('',*,*,#4263,.F.);
#5456=ORIENTED_EDGE('',*,*,#4268,.F.);
#5457=ORIENTED_EDGE('',*,*,#4269,.F.);
#5458=ORIENTED_EDGE('',*,*,#4270,.F.);
#5459=ORIENTED_EDGE('',*,*,#4266,.F.);
#5460=ORIENTED_EDGE('',*,*,#4271,.F.);
#5461=ORIENTED_EDGE('',*,*,#4272,.T.);
#5462=ORIENTED_EDGE('',*,*,#4273,.F.);
#5463=ORIENTED_EDGE('',*,*,#4272,.F.);
#5464=ORIENTED_EDGE('',*,*,#4185,.T.);
#5465=ORIENTED_EDGE('',*,*,#4274,.T.);
#5466=ORIENTED_EDGE('',*,*,#4275,.T.);
#5467=ORIENTED_EDGE('',*,*,#4276,.F.);
#5468=ORIENTED_EDGE('',*,*,#4162,.T.);
#5469=ORIENTED_EDGE('',*,*,#4277,.F.);
#5470=ORIENTED_EDGE('',*,*,#4278,.F.);
#5471=ORIENTED_EDGE('',*,*,#4279,.T.);
#5472=ORIENTED_EDGE('',*,*,#4213,.T.);
#5473=ORIENTED_EDGE('',*,*,#4280,.T.);
#5474=ORIENTED_EDGE('',*,*,#4278,.T.);
#5475=ORIENTED_EDGE('',*,*,#4281,.F.);
#5476=ORIENTED_EDGE('',*,*,#4190,.T.);
#5477=ORIENTED_EDGE('',*,*,#4282,.F.);
#5478=ORIENTED_EDGE('',*,*,#4283,.F.);
#5479=ORIENTED_EDGE('',*,*,#4284,.T.);
#5480=ORIENTED_EDGE('',*,*,#4241,.T.);
#5481=ORIENTED_EDGE('',*,*,#4285,.T.);
#5482=ORIENTED_EDGE('',*,*,#4283,.T.);
#5483=ORIENTED_EDGE('',*,*,#4286,.F.);
#5484=ORIENTED_EDGE('',*,*,#4218,.T.);
#5485=ORIENTED_EDGE('',*,*,#4287,.F.);
#5486=ORIENTED_EDGE('',*,*,#4288,.F.);
#5487=ORIENTED_EDGE('',*,*,#4289,.T.);
#5488=ORIENTED_EDGE('',*,*,#4269,.T.);
#5489=ORIENTED_EDGE('',*,*,#4290,.T.);
#5490=ORIENTED_EDGE('',*,*,#4288,.T.);
#5491=ORIENTED_EDGE('',*,*,#4291,.F.);
#5492=ORIENTED_EDGE('',*,*,#4246,.T.);
#5493=ORIENTED_EDGE('',*,*,#4292,.F.);
#5494=ORIENTED_EDGE('',*,*,#4275,.F.);
#5495=ORIENTED_EDGE('',*,*,#4293,.T.);
#5496=ORIENTED_EDGE('',*,*,#4161,.T.);
#5497=ORIENTED_EDGE('',*,*,#4165,.T.);
#5498=ORIENTED_EDGE('',*,*,#4168,.T.);
#5499=ORIENTED_EDGE('',*,*,#4171,.T.);
#5500=ORIENTED_EDGE('',*,*,#4174,.T.);
#5501=ORIENTED_EDGE('',*,*,#4177,.T.);
#5502=ORIENTED_EDGE('',*,*,#4180,.T.);
#5503=ORIENTED_EDGE('',*,*,#4183,.T.);
#5504=ORIENTED_EDGE('',*,*,#4186,.T.);
#5505=ORIENTED_EDGE('',*,*,#4276,.T.);
#5506=ORIENTED_EDGE('',*,*,#4292,.T.);
#5507=ORIENTED_EDGE('',*,*,#4245,.T.);
#5508=ORIENTED_EDGE('',*,*,#4249,.T.);
#5509=ORIENTED_EDGE('',*,*,#4252,.T.);
#5510=ORIENTED_EDGE('',*,*,#4255,.T.);
#5511=ORIENTED_EDGE('',*,*,#4258,.T.);
#5512=ORIENTED_EDGE('',*,*,#4261,.T.);
#5513=ORIENTED_EDGE('',*,*,#4264,.T.);
#5514=ORIENTED_EDGE('',*,*,#4267,.T.);
#5515=ORIENTED_EDGE('',*,*,#4270,.T.);
#5516=ORIENTED_EDGE('',*,*,#4291,.T.);
#5517=ORIENTED_EDGE('',*,*,#4287,.T.);
#5518=ORIENTED_EDGE('',*,*,#4217,.T.);
#5519=ORIENTED_EDGE('',*,*,#4221,.T.);
#5520=ORIENTED_EDGE('',*,*,#4224,.T.);
#5521=ORIENTED_EDGE('',*,*,#4227,.T.);
#5522=ORIENTED_EDGE('',*,*,#4230,.T.);
#5523=ORIENTED_EDGE('',*,*,#4233,.T.);
#5524=ORIENTED_EDGE('',*,*,#4236,.T.);
#5525=ORIENTED_EDGE('',*,*,#4239,.T.);
#5526=ORIENTED_EDGE('',*,*,#4242,.T.);
#5527=ORIENTED_EDGE('',*,*,#4286,.T.);
#5528=ORIENTED_EDGE('',*,*,#4282,.T.);
#5529=ORIENTED_EDGE('',*,*,#4189,.T.);
#5530=ORIENTED_EDGE('',*,*,#4193,.T.);
#5531=ORIENTED_EDGE('',*,*,#4196,.T.);
#5532=ORIENTED_EDGE('',*,*,#4199,.T.);
#5533=ORIENTED_EDGE('',*,*,#4202,.T.);
#5534=ORIENTED_EDGE('',*,*,#4205,.T.);
#5535=ORIENTED_EDGE('',*,*,#4208,.T.);
#5536=ORIENTED_EDGE('',*,*,#4211,.T.);
#5537=ORIENTED_EDGE('',*,*,#4214,.T.);
#5538=ORIENTED_EDGE('',*,*,#4281,.T.);
#5539=ORIENTED_EDGE('',*,*,#4277,.T.);
#5540=ORIENTED_EDGE('',*,*,#4273,.T.);
#5541=ORIENTED_EDGE('',*,*,#4159,.T.);
#5542=ORIENTED_EDGE('',*,*,#4279,.F.);
#5543=ORIENTED_EDGE('',*,*,#4280,.F.);
#5544=ORIENTED_EDGE('',*,*,#4212,.T.);
#5545=ORIENTED_EDGE('',*,*,#4209,.T.);
#5546=ORIENTED_EDGE('',*,*,#4206,.T.);
#5547=ORIENTED_EDGE('',*,*,#4203,.T.);
#5548=ORIENTED_EDGE('',*,*,#4200,.T.);
#5549=ORIENTED_EDGE('',*,*,#4197,.T.);
#5550=ORIENTED_EDGE('',*,*,#4194,.T.);
#5551=ORIENTED_EDGE('',*,*,#4191,.T.);
#5552=ORIENTED_EDGE('',*,*,#4187,.T.);
#5553=ORIENTED_EDGE('',*,*,#4284,.F.);
#5554=ORIENTED_EDGE('',*,*,#4285,.F.);
#5555=ORIENTED_EDGE('',*,*,#4240,.T.);
#5556=ORIENTED_EDGE('',*,*,#4237,.T.);
#5557=ORIENTED_EDGE('',*,*,#4234,.T.);
#5558=ORIENTED_EDGE('',*,*,#4231,.T.);
#5559=ORIENTED_EDGE('',*,*,#4228,.T.);
#5560=ORIENTED_EDGE('',*,*,#4225,.T.);
#5561=ORIENTED_EDGE('',*,*,#4222,.T.);
#5562=ORIENTED_EDGE('',*,*,#4219,.T.);
#5563=ORIENTED_EDGE('',*,*,#4215,.T.);
#5564=ORIENTED_EDGE('',*,*,#4289,.F.);
#5565=ORIENTED_EDGE('',*,*,#4290,.F.);
#5566=ORIENTED_EDGE('',*,*,#4268,.T.);
#5567=ORIENTED_EDGE('',*,*,#4265,.T.);
#5568=ORIENTED_EDGE('',*,*,#4262,.T.);
#5569=ORIENTED_EDGE('',*,*,#4259,.T.);
#5570=ORIENTED_EDGE('',*,*,#4256,.T.);
#5571=ORIENTED_EDGE('',*,*,#4253,.T.);
#5572=ORIENTED_EDGE('',*,*,#4250,.T.);
#5573=ORIENTED_EDGE('',*,*,#4247,.T.);
#5574=ORIENTED_EDGE('',*,*,#4243,.T.);
#5575=ORIENTED_EDGE('',*,*,#4293,.F.);
#5576=ORIENTED_EDGE('',*,*,#4274,.F.);
#5577=ORIENTED_EDGE('',*,*,#4184,.T.);
#5578=ORIENTED_EDGE('',*,*,#4181,.T.);
#5579=ORIENTED_EDGE('',*,*,#4178,.T.);
#5580=ORIENTED_EDGE('',*,*,#4175,.T.);
#5581=ORIENTED_EDGE('',*,*,#4172,.T.);
#5582=ORIENTED_EDGE('',*,*,#4169,.T.);
#5583=ORIENTED_EDGE('',*,*,#4166,.T.);
#5584=ORIENTED_EDGE('',*,*,#4163,.T.);
#5585=ORIENTED_EDGE('',*,*,#4271,.T.);
#6621=CYLINDRICAL_SURFACE('',#7789,0.21);
#6804=ADVANCED_FACE('',(#962),#619,.F.);
#6805=ADVANCED_FACE('',(#963),#620,.F.);
#6806=ADVANCED_FACE('',(#964),#621,.F.);
#6807=ADVANCED_FACE('',(#965),#622,.F.);
#6808=ADVANCED_FACE('',(#966),#623,.F.);
#6809=ADVANCED_FACE('',(#967),#624,.F.);
#6810=ADVANCED_FACE('',(#968),#625,.F.);
#6811=ADVANCED_FACE('',(#969),#626,.F.);
#6812=ADVANCED_FACE('',(#970),#627,.F.);
#6813=ADVANCED_FACE('',(#971),#628,.F.);
#6814=ADVANCED_FACE('',(#972),#629,.F.);
#6815=ADVANCED_FACE('',(#973),#630,.F.);
#6816=ADVANCED_FACE('',(#974),#631,.F.);
#6817=ADVANCED_FACE('',(#975),#632,.F.);
#6818=ADVANCED_FACE('',(#976),#633,.F.);
#6819=ADVANCED_FACE('',(#977),#634,.F.);
#6820=ADVANCED_FACE('',(#978),#635,.F.);
#6821=ADVANCED_FACE('',(#979),#636,.F.);
#6822=ADVANCED_FACE('',(#980),#637,.F.);
#6823=ADVANCED_FACE('',(#981),#638,.F.);
#6824=ADVANCED_FACE('',(#982),#639,.F.);
#6825=ADVANCED_FACE('',(#983),#640,.F.);
#6826=ADVANCED_FACE('',(#984),#641,.F.);
#6827=ADVANCED_FACE('',(#985),#642,.F.);
#6828=ADVANCED_FACE('',(#986),#643,.F.);
#6829=ADVANCED_FACE('',(#987),#644,.F.);
#6830=ADVANCED_FACE('',(#988),#645,.F.);
#6831=ADVANCED_FACE('',(#989),#646,.F.);
#6832=ADVANCED_FACE('',(#990),#647,.F.);
#6833=ADVANCED_FACE('',(#991),#648,.F.);
#6834=ADVANCED_FACE('',(#992),#649,.F.);
#6835=ADVANCED_FACE('',(#993),#650,.F.);
#6836=ADVANCED_FACE('',(#994),#651,.F.);
#6837=ADVANCED_FACE('',(#995),#652,.F.);
#6838=ADVANCED_FACE('',(#996),#653,.F.);
#6839=ADVANCED_FACE('',(#997),#654,.F.);
#6840=ADVANCED_FACE('',(#998),#6621,.F.);
#6841=ADVANCED_FACE('',(#999),#655,.T.);
#6842=ADVANCED_FACE('',(#1000),#656,.T.);
#6843=ADVANCED_FACE('',(#1001),#657,.T.);
#6844=ADVANCED_FACE('',(#1002),#658,.T.);
#6845=ADVANCED_FACE('',(#1003),#659,.T.);
#6846=ADVANCED_FACE('',(#1004),#660,.T.);
#6847=ADVANCED_FACE('',(#1005),#661,.T.);
#6848=ADVANCED_FACE('',(#1006),#662,.T.);
#6849=ADVANCED_FACE('',(#1007,#478),#663,.T.);
#6850=ADVANCED_FACE('',(#1008,#479),#664,.F.);
#7090=CLOSED_SHELL('',(#6804,#6805,#6806,#6807,#6808,#6809,#6810,#6811,
#6812,#6813,#6814,#6815,#6816,#6817,#6818,#6819,#6820,#6821,#6822,#6823,
#6824,#6825,#6826,#6827,#6828,#6829,#6830,#6831,#6832,#6833,#6834,#6835,
#6836,#6837,#6838,#6839,#6840,#6841,#6842,#6843,#6844,#6845,#6846,#6847,
#6848,#6849,#6850));
#7752=AXIS2_PLACEMENT_3D('',#13571,#8892,#8893);
#7753=AXIS2_PLACEMENT_3D('',#13572,#8894,#8895);
#7754=AXIS2_PLACEMENT_3D('',#13581,#8900,#8901);
#7755=AXIS2_PLACEMENT_3D('',#13587,#8905,#8906);
#7756=AXIS2_PLACEMENT_3D('',#13593,#8910,#8911);
#7757=AXIS2_PLACEMENT_3D('',#13599,#8915,#8916);
#7758=AXIS2_PLACEMENT_3D('',#13605,#8920,#8921);
#7759=AXIS2_PLACEMENT_3D('',#13611,#8925,#8926);
#7760=AXIS2_PLACEMENT_3D('',#13617,#8930,#8931);
#7761=AXIS2_PLACEMENT_3D('',#13623,#8935,#8936);
#7762=AXIS2_PLACEMENT_3D('',#13629,#8940,#8941);
#7763=AXIS2_PLACEMENT_3D('',#13638,#8946,#8947);
#7764=AXIS2_PLACEMENT_3D('',#13644,#8951,#8952);
#7765=AXIS2_PLACEMENT_3D('',#13650,#8956,#8957);
#7766=AXIS2_PLACEMENT_3D('',#13656,#8961,#8962);
#7767=AXIS2_PLACEMENT_3D('',#13662,#8966,#8967);
#7768=AXIS2_PLACEMENT_3D('',#13668,#8971,#8972);
#7769=AXIS2_PLACEMENT_3D('',#13674,#8976,#8977);
#7770=AXIS2_PLACEMENT_3D('',#13680,#8981,#8982);
#7771=AXIS2_PLACEMENT_3D('',#13686,#8986,#8987);
#7772=AXIS2_PLACEMENT_3D('',#13695,#8992,#8993);
#7773=AXIS2_PLACEMENT_3D('',#13701,#8997,#8998);
#7774=AXIS2_PLACEMENT_3D('',#13707,#9002,#9003);
#7775=AXIS2_PLACEMENT_3D('',#13713,#9007,#9008);
#7776=AXIS2_PLACEMENT_3D('',#13719,#9012,#9013);
#7777=AXIS2_PLACEMENT_3D('',#13725,#9017,#9018);
#7778=AXIS2_PLACEMENT_3D('',#13731,#9022,#9023);
#7779=AXIS2_PLACEMENT_3D('',#13737,#9027,#9028);
#7780=AXIS2_PLACEMENT_3D('',#13743,#9032,#9033);
#7781=AXIS2_PLACEMENT_3D('',#13752,#9038,#9039);
#7782=AXIS2_PLACEMENT_3D('',#13758,#9043,#9044);
#7783=AXIS2_PLACEMENT_3D('',#13764,#9048,#9049);
#7784=AXIS2_PLACEMENT_3D('',#13770,#9053,#9054);
#7785=AXIS2_PLACEMENT_3D('',#13776,#9058,#9059);
#7786=AXIS2_PLACEMENT_3D('',#13782,#9063,#9064);
#7787=AXIS2_PLACEMENT_3D('',#13788,#9068,#9069);
#7788=AXIS2_PLACEMENT_3D('',#13794,#9073,#9074);
#7789=AXIS2_PLACEMENT_3D('',#13800,#9078,#9079);
#7790=AXIS2_PLACEMENT_3D('',#13802,#9080,#9081);
#7791=AXIS2_PLACEMENT_3D('',#13805,#9083,#9084);
#7792=AXIS2_PLACEMENT_3D('',#13806,#9085,#9086);
#7793=AXIS2_PLACEMENT_3D('',#13812,#9090,#9091);
#7794=AXIS2_PLACEMENT_3D('',#13818,#9095,#9096);
#7795=AXIS2_PLACEMENT_3D('',#13821,#9099,#9100);
#7796=AXIS2_PLACEMENT_3D('',#13827,#9104,#9105);
#7797=AXIS2_PLACEMENT_3D('',#13830,#9108,#9109);
#7798=AXIS2_PLACEMENT_3D('',#13836,#9113,#9114);
#7799=AXIS2_PLACEMENT_3D('',#13839,#9117,#9118);
#7800=AXIS2_PLACEMENT_3D('',#13842,#9121,#9122);
#7801=AXIS2_PLACEMENT_3D('',#13843,#9123,#9124);
#8892=DIRECTION('axis',(0.,0.,1.));
#8893=DIRECTION('refdir',(1.,0.,0.));
#8894=DIRECTION('center_axis',(0.,0.,-1.));
#8895=DIRECTION('ref_axis',(0.,1.,0.));
#8896=DIRECTION('',(0.,1.,0.));
#8897=DIRECTION('',(1.,0.,0.));
#8898=DIRECTION('',(0.,-1.,0.));
#8899=DIRECTION('',(1.,0.,0.));
#8900=DIRECTION('center_axis',(0.,1.,-8.88178419700125E-16));
#8901=DIRECTION('ref_axis',(0.,8.88178419700125E-16,1.));
#8902=DIRECTION('',(0.,8.88178419700125E-16,1.));
#8903=DIRECTION('',(1.,0.,0.));
#8904=DIRECTION('',(0.,-8.88178419700125E-16,-1.));
#8905=DIRECTION('center_axis',(0.,-7.40148683083439E-16,-1.));
#8906=DIRECTION('ref_axis',(0.,1.,-7.40148683083439E-16));
#8907=DIRECTION('',(0.,1.,-7.40148683083439E-16));
#8908=DIRECTION('',(1.,0.,0.));
#8909=DIRECTION('',(0.,-1.,7.40148683083439E-16));
#8910=DIRECTION('center_axis',(0.,-0.707106781186547,-0.707106781186548));
#8911=DIRECTION('ref_axis',(0.,0.707106781186548,-0.707106781186547));
#8912=DIRECTION('',(0.,0.707106781186548,-0.707106781186547));
#8913=DIRECTION('',(1.,0.,0.));
#8914=DIRECTION('',(0.,-0.707106781186548,0.707106781186547));
#8915=DIRECTION('center_axis',(0.,-1.,2.77555756156289E-16));
#8916=DIRECTION('ref_axis',(0.,-2.77555756156289E-16,-1.));
#8917=DIRECTION('',(0.,-2.77555756156289E-16,-1.));
#8918=DIRECTION('',(1.,0.,0.));
#8919=DIRECTION('',(0.,2.77555756156289E-16,1.));
#8920=DIRECTION('center_axis',(0.,-0.707106781186547,0.707106781186548));
#8921=DIRECTION('ref_axis',(0.,-0.707106781186548,-0.707106781186547));
#8922=DIRECTION('',(0.,-0.707106781186548,-0.707106781186547));
#8923=DIRECTION('',(1.,0.,0.));
#8924=DIRECTION('',(0.,0.707106781186548,0.707106781186547));
#8925=DIRECTION('center_axis',(0.,7.40148683083438E-16,1.));
#8926=DIRECTION('ref_axis',(0.,-1.,7.40148683083438E-16));
#8927=DIRECTION('',(0.,-1.,7.40148683083438E-16));
#8928=DIRECTION('',(1.,0.,0.));
#8929=DIRECTION('',(0.,1.,-7.40148683083438E-16));
#8930=DIRECTION('center_axis',(0.,1.,-4.44089209850063E-16));
#8931=DIRECTION('ref_axis',(0.,4.44089209850063E-16,1.));
#8932=DIRECTION('',(0.,4.44089209850063E-16,1.));
#8933=DIRECTION('',(1.,0.,0.));
#8934=DIRECTION('',(0.,-4.44089209850063E-16,-1.));
#8935=DIRECTION('center_axis',(0.,2.41352831440251E-16,1.));
#8936=DIRECTION('ref_axis',(0.,-1.,2.41352831440251E-16));
#8937=DIRECTION('',(0.,-1.,2.41352831440251E-16));
#8938=DIRECTION('',(-1.,0.,0.));
#8939=DIRECTION('',(0.,1.,-2.41352831440251E-16));
#8940=DIRECTION('center_axis',(0.,-1.,2.41352831440251E-16));
#8941=DIRECTION('ref_axis',(0.,-2.41352831440251E-16,-1.));
#8942=DIRECTION('',(0.,-2.41352831440251E-16,-1.));
#8943=DIRECTION('',(1.,0.,0.));
#8944=DIRECTION('',(0.,2.41352831440251E-16,1.));
#8945=DIRECTION('',(1.,0.,0.));
#8946=DIRECTION('center_axis',(0.,0.,-1.));
#8947=DIRECTION('ref_axis',(0.,1.,0.));
#8948=DIRECTION('',(0.,1.,0.));
#8949=DIRECTION('',(1.,0.,0.));
#8950=DIRECTION('',(0.,-1.,0.));
#8951=DIRECTION('center_axis',(0.,-1.,0.));
#8952=DIRECTION('ref_axis',(0.,0.,-1.));
#8953=DIRECTION('',(0.,0.,-1.));
#8954=DIRECTION('',(1.,0.,0.));
#8955=DIRECTION('',(0.,0.,1.));
#8956=DIRECTION('center_axis',(0.,-0.707106781186547,0.707106781186548));
#8957=DIRECTION('ref_axis',(0.,-0.707106781186548,-0.707106781186547));
#8958=DIRECTION('',(0.,-0.707106781186548,-0.707106781186547));
#8959=DIRECTION('',(1.,0.,0.));
#8960=DIRECTION('',(0.,0.707106781186548,0.707106781186547));
#8961=DIRECTION('center_axis',(0.,0.,1.));
#8962=DIRECTION('ref_axis',(0.,-1.,0.));
#8963=DIRECTION('',(0.,-1.,0.));
#8964=DIRECTION('',(1.,0.,0.));
#8965=DIRECTION('',(0.,1.,0.));
#8966=DIRECTION('center_axis',(0.,0.707106781186548,0.707106781186547));
#8967=DIRECTION('ref_axis',(0.,-0.707106781186547,0.707106781186548));
#8968=DIRECTION('',(0.,-0.707106781186547,0.707106781186548));
#8969=DIRECTION('',(1.,0.,0.));
#8970=DIRECTION('',(0.,0.707106781186547,-0.707106781186548));
#8971=DIRECTION('center_axis',(0.,1.,0.));
#8972=DIRECTION('ref_axis',(0.,0.,1.));
#8973=DIRECTION('',(0.,0.,1.));
#8974=DIRECTION('',(1.,0.,0.));
#8975=DIRECTION('',(0.,0.,-1.));
#8976=DIRECTION('center_axis',(0.,0.,-1.));
#8977=DIRECTION('ref_axis',(0.,1.,0.));
#8978=DIRECTION('',(0.,1.,0.));
#8979=DIRECTION('',(1.,0.,0.));
#8980=DIRECTION('',(0.,-1.,0.));
#8981=DIRECTION('center_axis',(0.,1.,-2.41352831440251E-16));
#8982=DIRECTION('ref_axis',(0.,2.41352831440251E-16,1.));
#8983=DIRECTION('',(0.,2.41352831440251E-16,1.));
#8984=DIRECTION('',(-1.,0.,0.));
#8985=DIRECTION('',(0.,-2.41352831440251E-16,-1.));
#8986=DIRECTION('center_axis',(0.,0.,1.));
#8987=DIRECTION('ref_axis',(0.,-1.,0.));
#8988=DIRECTION('',(0.,-1.,0.));
#8989=DIRECTION('',(1.,0.,0.));
#8990=DIRECTION('',(0.,1.,0.));
#8991=DIRECTION('',(1.,0.,0.));
#8992=DIRECTION('center_axis',(0.,-1.,0.));
#8993=DIRECTION('ref_axis',(0.,0.,-1.));
#8994=DIRECTION('',(0.,0.,-1.));
#8995=DIRECTION('',(1.,0.,0.));
#8996=DIRECTION('',(0.,0.,1.));
#8997=DIRECTION('center_axis',(0.,0.,1.));
#8998=DIRECTION('ref_axis',(0.,-1.,0.));
#8999=DIRECTION('',(0.,-1.,0.));
#9000=DIRECTION('',(1.,0.,0.));
#9001=DIRECTION('',(0.,1.,0.));
#9002=DIRECTION('center_axis',(0.,0.707106781186548,0.707106781186548));
#9003=DIRECTION('ref_axis',(0.,-0.707106781186548,0.707106781186548));
#9004=DIRECTION('',(0.,-0.707106781186548,0.707106781186548));
#9005=DIRECTION('',(1.,0.,0.));
#9006=DIRECTION('',(0.,0.707106781186548,-0.707106781186548));
#9007=DIRECTION('center_axis',(0.,1.,0.));
#9008=DIRECTION('ref_axis',(0.,0.,1.));
#9009=DIRECTION('',(0.,0.,1.));
#9010=DIRECTION('',(1.,0.,0.));
#9011=DIRECTION('',(0.,0.,-1.));
#9012=DIRECTION('center_axis',(0.,0.707106781186548,-0.707106781186547));
#9013=DIRECTION('ref_axis',(0.,0.707106781186547,0.707106781186548));
#9014=DIRECTION('',(0.,0.707106781186547,0.707106781186548));
#9015=DIRECTION('',(1.,0.,0.));
#9016=DIRECTION('',(0.,-0.707106781186547,-0.707106781186548));
#9017=DIRECTION('center_axis',(0.,-7.40148683083438E-16,-1.));
#9018=DIRECTION('ref_axis',(0.,1.,-7.40148683083438E-16));
#9019=DIRECTION('',(0.,1.,-7.40148683083438E-16));
#9020=DIRECTION('',(1.,0.,0.));
#9021=DIRECTION('',(0.,-1.,7.40148683083438E-16));
#9022=DIRECTION('center_axis',(0.,-1.,0.));
#9023=DIRECTION('ref_axis',(0.,0.,-1.));
#9024=DIRECTION('',(0.,0.,-1.));
#9025=DIRECTION('',(1.,0.,0.));
#9026=DIRECTION('',(0.,0.,1.));
#9027=DIRECTION('center_axis',(0.,0.,-1.));
#9028=DIRECTION('ref_axis',(0.,1.,0.));
#9029=DIRECTION('',(0.,1.,0.));
#9030=DIRECTION('',(-1.,0.,0.));
#9031=DIRECTION('',(0.,-1.,0.));
#9032=DIRECTION('center_axis',(0.,1.,0.));
#9033=DIRECTION('ref_axis',(0.,0.,1.));
#9034=DIRECTION('',(0.,0.,1.));
#9035=DIRECTION('',(1.,0.,0.));
#9036=DIRECTION('',(0.,0.,-1.));
#9037=DIRECTION('',(1.,0.,0.));
#9038=DIRECTION('center_axis',(0.,0.,1.));
#9039=DIRECTION('ref_axis',(0.,-1.,0.));
#9040=DIRECTION('',(0.,-1.,0.));
#9041=DIRECTION('',(1.,0.,0.));
#9042=DIRECTION('',(0.,1.,0.));
#9043=DIRECTION('center_axis',(0.,1.,0.));
#9044=DIRECTION('ref_axis',(0.,0.,1.));
#9045=DIRECTION('',(0.,0.,1.));
#9046=DIRECTION('',(1.,0.,0.));
#9047=DIRECTION('',(0.,0.,-1.));
#9048=DIRECTION('center_axis',(0.,0.707106781186547,-0.707106781186548));
#9049=DIRECTION('ref_axis',(0.,0.707106781186548,0.707106781186547));
#9050=DIRECTION('',(0.,0.707106781186548,0.707106781186547));
#9051=DIRECTION('',(1.,0.,0.));
#9052=DIRECTION('',(0.,-0.707106781186548,-0.707106781186547));
#9053=DIRECTION('center_axis',(0.,0.,-1.));
#9054=DIRECTION('ref_axis',(0.,1.,0.));
#9055=DIRECTION('',(0.,1.,0.));
#9056=DIRECTION('',(1.,0.,0.));
#9057=DIRECTION('',(0.,-1.,0.));
#9058=DIRECTION('center_axis',(0.,-0.707106781186547,-0.707106781186548));
#9059=DIRECTION('ref_axis',(0.,0.707106781186548,-0.707106781186547));
#9060=DIRECTION('',(0.,0.707106781186548,-0.707106781186547));
#9061=DIRECTION('',(1.,0.,0.));
#9062=DIRECTION('',(0.,-0.707106781186548,0.707106781186547));
#9063=DIRECTION('center_axis',(0.,-1.,0.));
#9064=DIRECTION('ref_axis',(0.,0.,-1.));
#9065=DIRECTION('',(0.,0.,-1.));
#9066=DIRECTION('',(1.,0.,0.));
#9067=DIRECTION('',(0.,0.,1.));
#9068=DIRECTION('center_axis',(0.,0.,1.));
#9069=DIRECTION('ref_axis',(0.,-1.,0.));
#9070=DIRECTION('',(0.,-1.,0.));
#9071=DIRECTION('',(1.,0.,0.));
#9072=DIRECTION('',(0.,1.,0.));
#9073=DIRECTION('center_axis',(0.,-1.,0.));
#9074=DIRECTION('ref_axis',(0.,0.,-1.));
#9075=DIRECTION('',(0.,0.,-1.));
#9076=DIRECTION('',(-1.,0.,0.));
#9077=DIRECTION('',(0.,0.,1.));
#9078=DIRECTION('center_axis',(1.,0.,0.));
#9079=DIRECTION('ref_axis',(0.,0.,-1.));
#9080=DIRECTION('center_axis',(1.,0.,0.));
#9081=DIRECTION('ref_axis',(0.,0.,-1.));
#9082=DIRECTION('',(1.,0.,0.));
#9083=DIRECTION('center_axis',(-1.,0.,0.));
#9084=DIRECTION('ref_axis',(0.,0.,-1.));
#9085=DIRECTION('center_axis',(0.,1.,0.));
#9086=DIRECTION('ref_axis',(0.,0.,1.));
#9087=DIRECTION('',(0.,0.,1.));
#9088=DIRECTION('',(1.,0.,0.));
#9089=DIRECTION('',(0.,0.,1.));
#9090=DIRECTION('center_axis',(0.,1.,0.));
#9091=DIRECTION('ref_axis',(0.,0.,1.));
#9092=DIRECTION('',(0.,0.,1.));
#9093=DIRECTION('',(1.,0.,0.));
#9094=DIRECTION('',(0.,0.,1.));
#9095=DIRECTION('center_axis',(0.,0.,-1.));
#9096=DIRECTION('ref_axis',(0.,1.,0.));
#9097=DIRECTION('',(0.,1.,0.));
#9098=DIRECTION('',(0.,1.,0.));
#9099=DIRECTION('center_axis',(0.,0.,-1.));
#9100=DIRECTION('ref_axis',(0.,1.,0.));
#9101=DIRECTION('',(0.,1.,0.));
#9102=DIRECTION('',(1.,0.,0.));
#9103=DIRECTION('',(0.,1.,0.));
#9104=DIRECTION('center_axis',(0.,-1.,0.));
#9105=DIRECTION('ref_axis',(0.,0.,-1.));
#9106=DIRECTION('',(0.,0.,-1.));
#9107=DIRECTION('',(0.,0.,-1.));
#9108=DIRECTION('center_axis',(0.,-1.,0.));
#9109=DIRECTION('ref_axis',(0.,0.,-1.));
#9110=DIRECTION('',(0.,0.,-1.));
#9111=DIRECTION('',(1.,0.,0.));
#9112=DIRECTION('',(0.,0.,-1.));
#9113=DIRECTION('center_axis',(0.,0.,1.));
#9114=DIRECTION('ref_axis',(0.,-1.,0.));
#9115=DIRECTION('',(0.,-1.,0.));
#9116=DIRECTION('',(0.,-1.,0.));
#9117=DIRECTION('center_axis',(0.,0.,1.));
#9118=DIRECTION('ref_axis',(0.,-1.,0.));
#9119=DIRECTION('',(0.,-1.,0.));
#9120=DIRECTION('',(0.,-1.,0.));
#9121=DIRECTION('center_axis',(1.,0.,0.));
#9122=DIRECTION('ref_axis',(0.,0.,-1.));
#9123=DIRECTION('center_axis',(1.,0.,0.));
#9124=DIRECTION('ref_axis',(0.,0.,-1.));
#13571=CARTESIAN_POINT('',(0.,0.,0.));
#13572=CARTESIAN_POINT('Origin',(-0.1,0.82,-0.3));
#13573=CARTESIAN_POINT('',(0.,0.82,-0.3));
#13574=CARTESIAN_POINT('',(0.,1.,-0.3));
#13575=CARTESIAN_POINT('',(0.,0.41,-0.3));
#13576=CARTESIAN_POINT('',(40.,0.82,-0.3));
#13577=CARTESIAN_POINT('',(-0.1,0.82,-0.3));
#13578=CARTESIAN_POINT('',(40.,1.,-0.3));
#13579=CARTESIAN_POINT('',(40.,0.41,-0.3));
#13580=CARTESIAN_POINT('',(-0.05,1.,-0.3));
#13581=CARTESIAN_POINT('Origin',(-0.1,0.82,-0.55));
#13582=CARTESIAN_POINT('',(0.,0.82,-0.55));
#13583=CARTESIAN_POINT('',(0.,0.82,-0.275));
#13584=CARTESIAN_POINT('',(40.,0.82,-0.55));
#13585=CARTESIAN_POINT('',(-0.1,0.82,-0.55));
#13586=CARTESIAN_POINT('',(40.,0.82,-0.275));
#13587=CARTESIAN_POINT('Origin',(-0.1,0.67,-0.55));
#13588=CARTESIAN_POINT('',(0.,0.67,-0.55));
#13589=CARTESIAN_POINT('',(0.,0.335,-0.55));
#13590=CARTESIAN_POINT('',(40.,0.67,-0.55));
#13591=CARTESIAN_POINT('',(-0.1,0.67,-0.55));
#13592=CARTESIAN_POINT('',(40.,0.335,-0.55));
#13593=CARTESIAN_POINT('Origin',(-0.1,0.42,-0.3));
#13594=CARTESIAN_POINT('',(0.,0.42,-0.3));
#13595=CARTESIAN_POINT('',(0.,0.24,-0.12));
#13596=CARTESIAN_POINT('',(40.,0.42,-0.3));
#13597=CARTESIAN_POINT('',(-0.1,0.42,-0.3));
#13598=CARTESIAN_POINT('',(40.,0.24,-0.12));
#13599=CARTESIAN_POINT('Origin',(-0.1,0.42,0.3));
#13600=CARTESIAN_POINT('',(0.,0.42,0.3));
#13601=CARTESIAN_POINT('',(0.,0.42,0.15));
#13602=CARTESIAN_POINT('',(40.,0.42,0.3));
#13603=CARTESIAN_POINT('',(-0.1,0.42,0.3));
#13604=CARTESIAN_POINT('',(40.,0.42,0.15));
#13605=CARTESIAN_POINT('Origin',(-0.1,0.67,0.55));
#13606=CARTESIAN_POINT('',(0.,0.67,0.55));
#13607=CARTESIAN_POINT('',(6.93889390390723E-18,0.365,0.245));
#13608=CARTESIAN_POINT('',(40.,0.67,0.55));
#13609=CARTESIAN_POINT('',(-0.1,0.67,0.55));
#13610=CARTESIAN_POINT('',(40.,0.365,0.245));
#13611=CARTESIAN_POINT('Origin',(-0.1,0.82,0.55));
#13612=CARTESIAN_POINT('',(0.,0.82,0.55));
#13613=CARTESIAN_POINT('',(0.,0.41,0.55));
#13614=CARTESIAN_POINT('',(40.,0.82,0.55));
#13615=CARTESIAN_POINT('',(-0.1,0.82,0.55));
#13616=CARTESIAN_POINT('',(40.,0.41,0.55));
#13617=CARTESIAN_POINT('Origin',(-0.1,0.82,0.3));
#13618=CARTESIAN_POINT('',(0.,0.82,0.3));
#13619=CARTESIAN_POINT('',(0.,0.82,0.15));
#13620=CARTESIAN_POINT('',(40.,0.82,0.3));
#13621=CARTESIAN_POINT('',(-0.1,0.82,0.3));
#13622=CARTESIAN_POINT('',(40.,0.82,0.15));
#13623=CARTESIAN_POINT('Origin',(-0.1,1.05,0.3));
#13624=CARTESIAN_POINT('',(0.,1.,0.3));
#13625=CARTESIAN_POINT('',(0.,0.525,0.3));
#13626=CARTESIAN_POINT('',(40.,1.,0.3));
#13627=CARTESIAN_POINT('',(-0.05,1.,0.3));
#13628=CARTESIAN_POINT('',(40.,0.525,0.3));
#13629=CARTESIAN_POINT('Origin',(-0.1,-0.3,-0.82));
#13630=CARTESIAN_POINT('',(0.,-0.3,-0.82));
#13631=CARTESIAN_POINT('',(0.,-0.3,-1.));
#13632=CARTESIAN_POINT('',(0.,-0.3,-0.41));
#13633=CARTESIAN_POINT('',(40.,-0.3,-0.82));
#13634=CARTESIAN_POINT('',(-0.1,-0.3,-0.82));
#13635=CARTESIAN_POINT('',(40.,-0.3,-1.));
#13636=CARTESIAN_POINT('',(40.,-0.3,-0.41));
#13637=CARTESIAN_POINT('',(-0.05,-0.3,-1.));
#13638=CARTESIAN_POINT('Origin',(-0.1,-0.55,-0.82));
#13639=CARTESIAN_POINT('',(0.,-0.55,-0.82));
#13640=CARTESIAN_POINT('',(0.,-0.275,-0.82));
#13641=CARTESIAN_POINT('',(40.,-0.55,-0.82));
#13642=CARTESIAN_POINT('',(-0.1,-0.55,-0.82));
#13643=CARTESIAN_POINT('',(40.,-0.275,-0.82));
#13644=CARTESIAN_POINT('Origin',(-0.1,-0.55,-0.67));
#13645=CARTESIAN_POINT('',(0.,-0.55,-0.67));
#13646=CARTESIAN_POINT('',(0.,-0.55,-0.335));
#13647=CARTESIAN_POINT('',(40.,-0.55,-0.67));
#13648=CARTESIAN_POINT('',(-0.1,-0.55,-0.67));
#13649=CARTESIAN_POINT('',(40.,-0.55,-0.335));
#13650=CARTESIAN_POINT('Origin',(-0.1,-0.3,-0.42));
#13651=CARTESIAN_POINT('',(0.,-0.3,-0.42));
#13652=CARTESIAN_POINT('',(0.,-0.12,-0.24));
#13653=CARTESIAN_POINT('',(40.,-0.3,-0.42));
#13654=CARTESIAN_POINT('',(-0.1,-0.3,-0.42));
#13655=CARTESIAN_POINT('',(40.,-0.12,-0.24));
#13656=CARTESIAN_POINT('Origin',(-0.1,0.3,-0.42));
#13657=CARTESIAN_POINT('',(0.,0.3,-0.42));
#13658=CARTESIAN_POINT('',(0.,0.15,-0.42));
#13659=CARTESIAN_POINT('',(40.,0.3,-0.42));
#13660=CARTESIAN_POINT('',(-0.1,0.3,-0.42));
#13661=CARTESIAN_POINT('',(40.,0.15,-0.42));
#13662=CARTESIAN_POINT('Origin',(-0.1,0.55,-0.67));
#13663=CARTESIAN_POINT('',(0.,0.55,-0.67));
#13664=CARTESIAN_POINT('',(0.,0.245,-0.365));
#13665=CARTESIAN_POINT('',(40.,0.55,-0.67));
#13666=CARTESIAN_POINT('',(-0.1,0.55,-0.67));
#13667=CARTESIAN_POINT('',(40.,0.245,-0.365));
#13668=CARTESIAN_POINT('Origin',(-0.1,0.55,-0.82));
#13669=CARTESIAN_POINT('',(0.,0.55,-0.82));
#13670=CARTESIAN_POINT('',(0.,0.55,-0.41));
#13671=CARTESIAN_POINT('',(40.,0.55,-0.82));
#13672=CARTESIAN_POINT('',(-0.1,0.55,-0.82));
#13673=CARTESIAN_POINT('',(40.,0.55,-0.41));
#13674=CARTESIAN_POINT('Origin',(-0.1,0.3,-0.82));
#13675=CARTESIAN_POINT('',(0.,0.3,-0.82));
#13676=CARTESIAN_POINT('',(0.,0.15,-0.82));
#13677=CARTESIAN_POINT('',(40.,0.3,-0.82));
#13678=CARTESIAN_POINT('',(-0.1,0.3,-0.82));
#13679=CARTESIAN_POINT('',(40.,0.15,-0.82));
#13680=CARTESIAN_POINT('Origin',(-0.1,0.3,-1.05));
#13681=CARTESIAN_POINT('',(0.,0.3,-1.));
#13682=CARTESIAN_POINT('',(0.,0.3,-0.525));
#13683=CARTESIAN_POINT('',(40.,0.3,-1.));
#13684=CARTESIAN_POINT('',(-0.05,0.3,-1.));
#13685=CARTESIAN_POINT('',(40.,0.3,-0.525));
#13686=CARTESIAN_POINT('Origin',(-0.1,-0.82,0.3));
#13687=CARTESIAN_POINT('',(0.,-0.82,0.3));
#13688=CARTESIAN_POINT('',(0.,-1.,0.3));
#13689=CARTESIAN_POINT('',(0.,-0.41,0.3));
#13690=CARTESIAN_POINT('',(40.,-0.82,0.3));
#13691=CARTESIAN_POINT('',(-0.1,-0.82,0.3));
#13692=CARTESIAN_POINT('',(40.,-1.,0.3));
#13693=CARTESIAN_POINT('',(40.,-0.41,0.3));
#13694=CARTESIAN_POINT('',(-0.05,-1.,0.3));
#13695=CARTESIAN_POINT('Origin',(-0.1,-0.82,0.55));
#13696=CARTESIAN_POINT('',(0.,-0.82,0.55));
#13697=CARTESIAN_POINT('',(0.,-0.82,0.275));
#13698=CARTESIAN_POINT('',(40.,-0.82,0.55));
#13699=CARTESIAN_POINT('',(-0.1,-0.82,0.55));
#13700=CARTESIAN_POINT('',(40.,-0.82,0.275));
#13701=CARTESIAN_POINT('Origin',(-0.1,-0.67,0.55));
#13702=CARTESIAN_POINT('',(0.,-0.67,0.55));
#13703=CARTESIAN_POINT('',(0.,-0.335,0.55));
#13704=CARTESIAN_POINT('',(40.,-0.67,0.55));
#13705=CARTESIAN_POINT('',(-0.1,-0.67,0.55));
#13706=CARTESIAN_POINT('',(40.,-0.335,0.55));
#13707=CARTESIAN_POINT('Origin',(-0.1,-0.42,0.3));
#13708=CARTESIAN_POINT('',(0.,-0.42,0.3));
#13709=CARTESIAN_POINT('',(-6.93889390390723E-18,-0.24,0.12));
#13710=CARTESIAN_POINT('',(40.,-0.42,0.3));
#13711=CARTESIAN_POINT('',(-0.1,-0.42,0.3));
#13712=CARTESIAN_POINT('',(40.,-0.24,0.12));
#13713=CARTESIAN_POINT('Origin',(-0.1,-0.42,-0.3));
#13714=CARTESIAN_POINT('',(0.,-0.42,-0.3));
#13715=CARTESIAN_POINT('',(0.,-0.42,-0.15));
#13716=CARTESIAN_POINT('',(40.,-0.42,-0.3));
#13717=CARTESIAN_POINT('',(-0.1,-0.42,-0.3));
#13718=CARTESIAN_POINT('',(40.,-0.42,-0.15));
#13719=CARTESIAN_POINT('Origin',(-0.1,-0.67,-0.55));
#13720=CARTESIAN_POINT('',(0.,-0.67,-0.55));
#13721=CARTESIAN_POINT('',(0.,-0.365,-0.245));
#13722=CARTESIAN_POINT('',(40.,-0.67,-0.55));
#13723=CARTESIAN_POINT('',(-0.1,-0.67,-0.55));
#13724=CARTESIAN_POINT('',(40.,-0.365,-0.245));
#13725=CARTESIAN_POINT('Origin',(-0.1,-0.82,-0.55));
#13726=CARTESIAN_POINT('',(0.,-0.82,-0.55));
#13727=CARTESIAN_POINT('',(0.,-0.41,-0.55));
#13728=CARTESIAN_POINT('',(40.,-0.82,-0.55));
#13729=CARTESIAN_POINT('',(-0.1,-0.82,-0.55));
#13730=CARTESIAN_POINT('',(40.,-0.41,-0.55));
#13731=CARTESIAN_POINT('Origin',(-0.1,-0.82,-0.3));
#13732=CARTESIAN_POINT('',(0.,-0.82,-0.3));
#13733=CARTESIAN_POINT('',(0.,-0.82,-0.15));
#13734=CARTESIAN_POINT('',(40.,-0.82,-0.3));
#13735=CARTESIAN_POINT('',(-0.1,-0.82,-0.3));
#13736=CARTESIAN_POINT('',(40.,-0.82,-0.15));
#13737=CARTESIAN_POINT('Origin',(-0.1,-1.05,-0.3));
#13738=CARTESIAN_POINT('',(0.,-1.,-0.3));
#13739=CARTESIAN_POINT('',(0.,-0.525,-0.3));
#13740=CARTESIAN_POINT('',(40.,-1.,-0.3));
#13741=CARTESIAN_POINT('',(-0.05,-1.,-0.3));
#13742=CARTESIAN_POINT('',(40.,-0.525,-0.3));
#13743=CARTESIAN_POINT('Origin',(-0.1,0.3,0.82));
#13744=CARTESIAN_POINT('',(0.,0.3,0.82));
#13745=CARTESIAN_POINT('',(0.,0.3,1.));
#13746=CARTESIAN_POINT('',(0.,0.3,0.41));
#13747=CARTESIAN_POINT('',(40.,0.3,0.82));
#13748=CARTESIAN_POINT('',(-0.1,0.3,0.82));
#13749=CARTESIAN_POINT('',(40.,0.3,1.));
#13750=CARTESIAN_POINT('',(40.,0.3,0.41));
#13751=CARTESIAN_POINT('',(-0.05,0.3,1.));
#13752=CARTESIAN_POINT('Origin',(-0.1,0.55,0.82));
#13753=CARTESIAN_POINT('',(0.,0.55,0.82));
#13754=CARTESIAN_POINT('',(0.,0.275,0.82));
#13755=CARTESIAN_POINT('',(40.,0.55,0.82));
#13756=CARTESIAN_POINT('',(-0.1,0.55,0.82));
#13757=CARTESIAN_POINT('',(40.,0.275,0.82));
#13758=CARTESIAN_POINT('Origin',(-0.1,0.55,0.67));
#13759=CARTESIAN_POINT('',(0.,0.55,0.67));
#13760=CARTESIAN_POINT('',(0.,0.55,0.335));
#13761=CARTESIAN_POINT('',(40.,0.55,0.67));
#13762=CARTESIAN_POINT('',(-0.1,0.55,0.67));
#13763=CARTESIAN_POINT('',(40.,0.55,0.335));
#13764=CARTESIAN_POINT('Origin',(-0.1,0.3,0.42));
#13765=CARTESIAN_POINT('',(0.,0.3,0.42));
#13766=CARTESIAN_POINT('',(6.93889390390723E-18,0.12,0.24));
#13767=CARTESIAN_POINT('',(40.,0.3,0.42));
#13768=CARTESIAN_POINT('',(-0.1,0.3,0.42));
#13769=CARTESIAN_POINT('',(40.,0.12,0.24));
#13770=CARTESIAN_POINT('Origin',(-0.1,-0.3,0.42));
#13771=CARTESIAN_POINT('',(0.,-0.3,0.42));
#13772=CARTESIAN_POINT('',(0.,-0.15,0.42));
#13773=CARTESIAN_POINT('',(40.,-0.3,0.42));
#13774=CARTESIAN_POINT('',(-0.1,-0.3,0.42));
#13775=CARTESIAN_POINT('',(40.,-0.15,0.42));
#13776=CARTESIAN_POINT('Origin',(-0.1,-0.55,0.67));
#13777=CARTESIAN_POINT('',(0.,-0.55,0.67));
#13778=CARTESIAN_POINT('',(6.93889390390723E-18,-0.245,0.365));
#13779=CARTESIAN_POINT('',(40.,-0.55,0.67));
#13780=CARTESIAN_POINT('',(-0.1,-0.55,0.67));
#13781=CARTESIAN_POINT('',(40.,-0.245,0.365));
#13782=CARTESIAN_POINT('Origin',(-0.1,-0.55,0.82));
#13783=CARTESIAN_POINT('',(0.,-0.55,0.82));
#13784=CARTESIAN_POINT('',(0.,-0.55,0.41));
#13785=CARTESIAN_POINT('',(40.,-0.55,0.82));
#13786=CARTESIAN_POINT('',(-0.1,-0.55,0.82));
#13787=CARTESIAN_POINT('',(40.,-0.55,0.41));
#13788=CARTESIAN_POINT('Origin',(-0.1,-0.3,0.82));
#13789=CARTESIAN_POINT('',(0.,-0.3,0.82));
#13790=CARTESIAN_POINT('',(0.,-0.15,0.82));
#13791=CARTESIAN_POINT('',(40.,-0.3,0.82));
#13792=CARTESIAN_POINT('',(-0.1,-0.3,0.82));
#13793=CARTESIAN_POINT('',(40.,-0.15,0.82));
#13794=CARTESIAN_POINT('Origin',(-0.1,-0.3,1.05));
#13795=CARTESIAN_POINT('',(0.,-0.3,1.));
#13796=CARTESIAN_POINT('',(0.,-0.3,0.525));
#13797=CARTESIAN_POINT('',(40.,-0.3,1.));
#13798=CARTESIAN_POINT('',(-0.05,-0.3,1.));
#13799=CARTESIAN_POINT('',(40.,-0.3,0.525));
#13800=CARTESIAN_POINT('Origin',(-0.1,0.,0.));
#13801=CARTESIAN_POINT('',(0.,-2.57175827820944E-17,0.21));
#13802=CARTESIAN_POINT('Origin',(0.,0.,0.));
#13803=CARTESIAN_POINT('',(40.,2.57175827820944E-17,0.21));
#13804=CARTESIAN_POINT('',(-0.1,-2.57175827820944E-17,0.21));
#13805=CARTESIAN_POINT('Origin',(40.,0.,0.));
#13806=CARTESIAN_POINT('Origin',(0.,1.,-1.));
#13807=CARTESIAN_POINT('',(0.,1.,1.));
#13808=CARTESIAN_POINT('',(0.,1.,-1.));
#13809=CARTESIAN_POINT('',(40.,1.,1.));
#13810=CARTESIAN_POINT('',(0.,1.,1.));
#13811=CARTESIAN_POINT('',(40.,1.,-1.));
#13812=CARTESIAN_POINT('Origin',(0.,1.,-1.));
#13813=CARTESIAN_POINT('',(40.,1.,-1.));
#13814=CARTESIAN_POINT('',(40.,1.,-1.));
#13815=CARTESIAN_POINT('',(0.,1.,-1.));
#13816=CARTESIAN_POINT('',(0.,1.,-1.));
#13817=CARTESIAN_POINT('',(0.,1.,-1.));
#13818=CARTESIAN_POINT('Origin',(0.,-1.,-1.));
#13819=CARTESIAN_POINT('',(0.,-1.,-1.));
#13820=CARTESIAN_POINT('',(40.,-1.,-1.));
#13821=CARTESIAN_POINT('Origin',(0.,-1.,-1.));
#13822=CARTESIAN_POINT('',(40.,-1.,-1.));
#13823=CARTESIAN_POINT('',(40.,-1.,-1.));
#13824=CARTESIAN_POINT('',(0.,-1.,-1.));
#13825=CARTESIAN_POINT('',(0.,-1.,-1.));
#13826=CARTESIAN_POINT('',(0.,-1.,-1.));
#13827=CARTESIAN_POINT('Origin',(0.,-1.,1.));
#13828=CARTESIAN_POINT('',(0.,-1.,1.));
#13829=CARTESIAN_POINT('',(40.,-1.,1.));
#13830=CARTESIAN_POINT('Origin',(0.,-1.,1.));
#13831=CARTESIAN_POINT('',(40.,-1.,1.));
#13832=CARTESIAN_POINT('',(40.,-1.,1.));
#13833=CARTESIAN_POINT('',(0.,-1.,1.));
#13834=CARTESIAN_POINT('',(0.,-1.,1.));
#13835=CARTESIAN_POINT('',(0.,-1.,1.));
#13836=CARTESIAN_POINT('Origin',(0.,1.,1.));
#13837=CARTESIAN_POINT('',(0.,1.,1.));
#13838=CARTESIAN_POINT('',(40.,1.,1.));
#13839=CARTESIAN_POINT('Origin',(0.,1.,1.));
#13840=CARTESIAN_POINT('',(40.,1.,1.));
#13841=CARTESIAN_POINT('',(0.,1.,1.));
#13842=CARTESIAN_POINT('Origin',(40.,0.,0.));
#13843=CARTESIAN_POINT('Origin',(0.,0.,0.));
#14980=UNCERTAINTY_MEASURE_WITH_UNIT(LENGTH_MEASURE(0.001),#15041,
'DISTANCE_ACCURACY_VALUE',
'Maximum model space distance between geometric entities at asserted c
onnectivities');
#15000=UNCERTAINTY_MEASURE_WITH_UNIT(LENGTH_MEASURE(0.001),#15041,
'DISTANCE_ACCURACY_VALUE',
'Maximum model space distance between geometric entities at asserted c
onnectivities');
#15020=(
GEOMETRIC_REPRESENTATION_CONTEXT(3)
GLOBAL_UNCERTAINTY_ASSIGNED_CONTEXT((#14980))
GLOBAL_UNIT_ASSIGNED_CONTEXT((#15041,#15043,#15044))
REPRESENTATION_CONTEXT('','3D')
);
#15040=(
GEOMETRIC_REPRESENTATION_CONTEXT(3)
GLOBAL_UNCERTAINTY_ASSIGNED_CONTEXT((#15000))
GLOBAL_UNIT_ASSIGNED_CONTEXT((#15041,#15043,#15044))
REPRESENTATION_CONTEXT('','3D')
);
#15041=(
LENGTH_UNIT()
NAMED_UNIT(*)
SI_UNIT(.CENTI.,.METRE.)
);
#15043=(
NAMED_UNIT(*)
PLANE_ANGLE_UNIT()
SI_UNIT($,.RADIAN.)
);
#15044=(
NAMED_UNIT(*)
SI_UNIT($,.STERADIAN.)
SOLID_ANGLE_UNIT()
);
#15064=SHAPE_DEFINITION_REPRESENTATION(#15103,#15201);
#15103=PRODUCT_DEFINITION_SHAPE('',$,#15241);
#15201=SHAPE_REPRESENTATION('',(#7752),#15020);
#15221=PRODUCT_DEFINITION_CONTEXT('part definition',#15340,'design');
#15241=PRODUCT_DEFINITION('Slotted Extrusion - 20 x 20 x 400 mm',
'Slotted Extrusion - 20 x 20 x 400 mm',#15280,#15221);
#15280=PRODUCT_DEFINITION_FORMATION('',$,#15361);
#15340=APPLICATION_CONTEXT(
'Core Data for Automotive Mechanical Design Process');
#15341=PRODUCT_CONTEXT('part definition',#15340,'mechanical');
#15361=PRODUCT('Slotted Extrusion - 20 x 20 x 400 mm',
'Slotted Extrusion - 20 x 20 x 400 mm',
'Slotted Extrusion - 20 x 20 x 400 mm',(#15341));
#15437=COLOUR_RGB('Light Blue',0.38,0.62,0.78);
#15438=FILL_AREA_STYLE_COLOUR('',#15437);
#15439=FILL_AREA_STYLE('',(#15438));
#15440=SURFACE_STYLE_FILL_AREA(#15439);
#15441=SURFACE_SIDE_STYLE('',(#15440));
#15442=SURFACE_STYLE_USAGE(.BOTH.,#15441);
#15443=PRESENTATION_STYLE_ASSIGNMENT((#15442));
ENDSEC;
END-ISO-10303-21;
